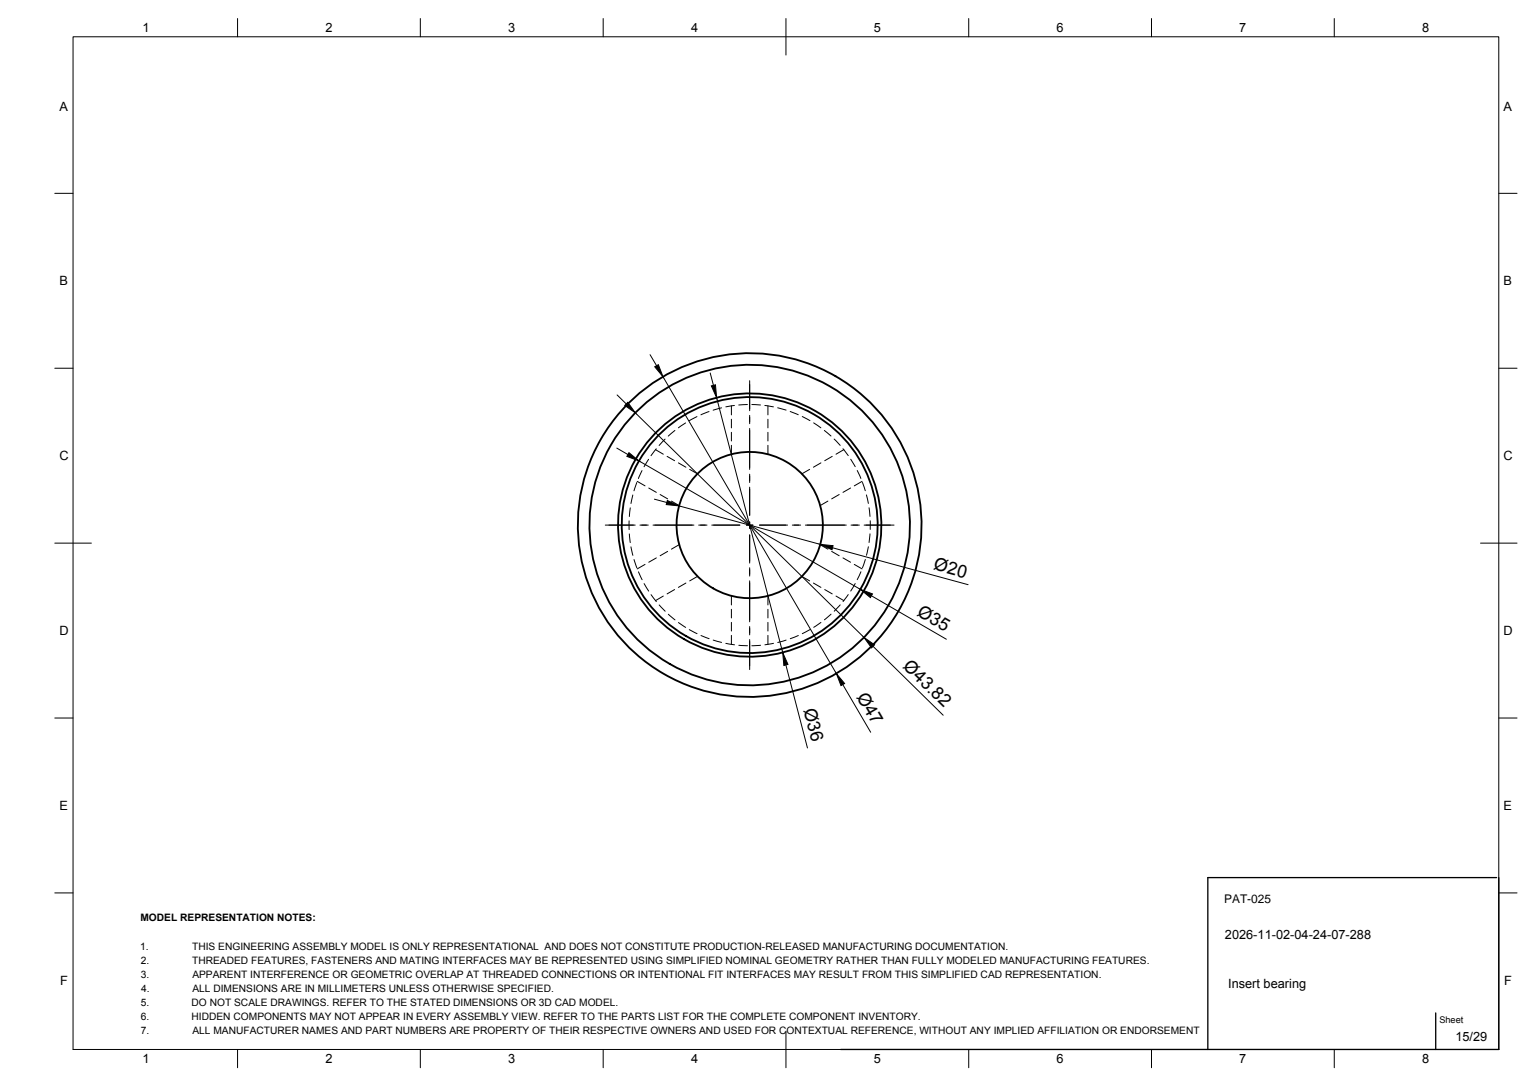
ISO-10303-21;
HEADER;
/* Generated by software containing ST-Developer
 * from STEP Tools, Inc. (www.steptools.com) 
 */

FILE_DESCRIPTION(
/* description */ ('Counter shaft with two pulleys and keyed hub'),
/* implementation_level */ '2;1');

FILE_NAME(
/* name */ 'Insert bearing.step',
/* time_stamp */ '2026-10-27T10:46:10-07:00',
/* author */ (''),
/* organization */ (''),
/* preprocessor_version */ 'ST-DEVELOPER v20.2',
/* originating_system */ 'Autodesk Translation Framework v15.17.0.0',
/* authorisation */ '');

FILE_SCHEMA (('AUTOMOTIVE_DESIGN { 1 0 10303 214 3 1 1 }'));
ENDSEC;

DATA;
#10=MECHANICAL_DESIGN_GEOMETRIC_PRESENTATION_REPRESENTATION('',(#298,#299),#10821);
#184=B_SPLINE_CURVE_WITH_KNOTS('',3,(#8629,#8630,#8631,#8632,#8633,#8634,
#8635,#8636,#8637,#8638),.UNSPECIFIED.,.F.,.F.,(4,2,2,2,4),(1.13193471301885,
1.22626174930539,1.32058878559194,1.41491753480854,1.50924628402513),
 .UNSPECIFIED.);
#185=B_SPLINE_CURVE_WITH_KNOTS('',3,(#8640,#8641,#8642,#8643,#8644,#8645,
#8646,#8647,#8648,#8649,#8650,#8651,#8652,#8653,#8654,#8655,#8656,#8657),
 .UNSPECIFIED.,.F.,.F.,(4,2,2,2,2,2,2,2,4),(0.377311571006283,0.471638607292829,
0.565965643579376,0.66029439279597,0.754623142012565,0.84895189122916,0.943280640445754,
1.0376076767323,1.13193471301885),.UNSPECIFIED.);
#186=B_SPLINE_CURVE_WITH_KNOTS('',3,(#8658,#8659,#8660,#8661,#8662,#8663,
#8664,#8665,#8666,#8667),.UNSPECIFIED.,.F.,.F.,(4,2,2,2,4),(1.50924628402513,
1.60357503324173,1.69790378245832,1.79223081874487,1.88655785503141),
 .UNSPECIFIED.);
#187=B_SPLINE_CURVE_WITH_KNOTS('',3,(#8670,#8671,#8672,#8673,#8674,#8675,
#8676,#8677,#8678,#8679,#8680,#8681,#8682,#8683,#8684,#8685,#8686,#8687,
#8688,#8689,#8690,#8691,#8692,#8693,#8694,#8695,#8696,#8697,#8698,#8699,
#8700,#8701,#8702,#8703),.UNSPECIFIED.,.T.,.F.,(4,2,2,2,2,2,2,2,2,2,2,2,
2,2,2,2,4),(0.,0.0946120580087934,0.189224116017587,0.283822945575014,0.378421775132442,
0.47302060468987,0.567619434247297,0.662231492256091,0.756843550264884,
0.851455608273677,0.94606766628247,1.0406664958399,1.13526532539733,1.22986415495475,
1.32446298451218,1.41907504252097,1.51368710052977),.UNSPECIFIED.);
#188=B_SPLINE_CURVE_WITH_KNOTS('',3,(#8706,#8707,#8708,#8709,#8710,#8711,
#8712,#8713,#8714,#8715,#8716,#8717,#8718,#8719,#8720,#8721,#8722,#8723,
#8724,#8725,#8726,#8727,#8728,#8729,#8730,#8731,#8732,#8733,#8734,#8735,
#8736,#8737,#8738,#8739),.UNSPECIFIED.,.T.,.F.,(4,2,2,2,2,2,2,2,2,2,2,2,
2,2,2,2,4),(0.,0.0946120580087934,0.189224116017587,0.283822945575014,0.378421775132442,
0.47302060468987,0.567619434247297,0.66223149225609,0.756843550264884,0.851455608273677,
0.94606766628247,1.0406664958399,1.13526532539733,1.22986415495475,1.32446298451218,
1.41907504252097,1.51368710052977),.UNSPECIFIED.);
#189=B_SPLINE_CURVE_WITH_KNOTS('',3,(#8743,#8744,#8745,#8746,#8747,#8748,
#8749,#8750,#8751,#8752),.UNSPECIFIED.,.F.,.F.,(4,2,2,2,4),(1.13193471301885,
1.22626174930539,1.32058878559194,1.41491753480854,1.50924628402513),
 .UNSPECIFIED.);
#190=B_SPLINE_CURVE_WITH_KNOTS('',3,(#8754,#8755,#8756,#8757,#8758,#8759,
#8760,#8761,#8762,#8763,#8764,#8765,#8766,#8767,#8768,#8769,#8770,#8771),
 .UNSPECIFIED.,.F.,.F.,(4,2,2,2,2,2,2,2,4),(0.377311571006283,0.47163860729283,
0.565965643579376,0.660294392795971,0.754623142012565,0.84895189122916,
0.943280640445755,1.0376076767323,1.13193471301885),.UNSPECIFIED.);
#191=B_SPLINE_CURVE_WITH_KNOTS('',3,(#8772,#8773,#8774,#8775,#8776,#8777,
#8778,#8779,#8780,#8781),.UNSPECIFIED.,.F.,.F.,(4,2,2,2,4),(1.50924628402513,
1.60357503324173,1.69790378245832,1.79223081874487,1.88655785503141),
 .UNSPECIFIED.);
#192=B_SPLINE_CURVE_WITH_KNOTS('',3,(#8790,#8791,#8792,#8793,#8794,#8795,
#8796,#8797,#8798,#8799,#8800,#8801,#8802,#8803,#8804,#8805,#8806,#8807),
 .UNSPECIFIED.,.F.,.F.,(4,2,2,2,2,2,2,2,4),(0.377311571006282,0.471638607292829,
0.565965643579376,0.660294392795971,0.754623142012565,0.84895189122916,
0.943280640445754,1.0376076767323,1.13193471301885),.UNSPECIFIED.);
#193=B_SPLINE_CURVE_WITH_KNOTS('',3,(#8809,#8810,#8811,#8812,#8813,#8814,
#8815,#8816,#8817,#8818),.UNSPECIFIED.,.F.,.F.,(4,2,2,2,4),(1.13193471301885,
1.22626174930539,1.32058878559194,1.41491753480854,1.50924628402513),
 .UNSPECIFIED.);
#194=B_SPLINE_CURVE_WITH_KNOTS('',3,(#8819,#8820,#8821,#8822,#8823,#8824,
#8825,#8826,#8827,#8828),.UNSPECIFIED.,.F.,.F.,(4,2,2,2,4),(1.50924628402513,
1.60357503324172,1.69790378245832,1.79223081874487,1.88655785503141),
 .UNSPECIFIED.);
#195=B_SPLINE_CURVE_WITH_KNOTS('',3,(#8831,#8832,#8833,#8834,#8835,#8836,
#8837,#8838,#8839,#8840,#8841,#8842,#8843,#8844,#8845,#8846,#8847,#8848),
 .UNSPECIFIED.,.F.,.F.,(4,2,2,2,2,2,2,2,4),(0.377311571006283,0.47163860729283,
0.565965643579376,0.660294392795971,0.754623142012565,0.84895189122916,
0.943280640445754,1.0376076767323,1.13193471301885),.UNSPECIFIED.);
#196=B_SPLINE_CURVE_WITH_KNOTS('',3,(#8850,#8851,#8852,#8853,#8854,#8855,
#8856,#8857,#8858,#8859),.UNSPECIFIED.,.F.,.F.,(4,2,2,2,4),(1.13193471301885,
1.22626174930539,1.32058878559194,1.41491753480854,1.50924628402513),
 .UNSPECIFIED.);
#197=B_SPLINE_CURVE_WITH_KNOTS('',3,(#8860,#8861,#8862,#8863,#8864,#8865,
#8866,#8867,#8868,#8869),.UNSPECIFIED.,.F.,.F.,(4,2,2,2,4),(1.50924628402513,
1.60357503324173,1.69790378245832,1.79223081874487,1.88655785503141),
 .UNSPECIFIED.);
#198=B_SPLINE_CURVE_WITH_KNOTS('',3,(#8872,#8873,#8874,#8875,#8876,#8877,
#8878,#8879,#8880,#8881,#8882,#8883,#8884,#8885,#8886,#8887,#8888,#8889),
 .UNSPECIFIED.,.F.,.F.,(4,2,2,2,2,2,2,2,4),(0.377311571006282,0.471638607292829,
0.565965643579376,0.66029439279597,0.754623142012565,0.84895189122916,0.943280640445754,
1.0376076767323,1.13193471301885),.UNSPECIFIED.);
#199=B_SPLINE_CURVE_WITH_KNOTS('',3,(#8891,#8892,#8893,#8894,#8895,#8896,
#8897,#8898,#8899,#8900),.UNSPECIFIED.,.F.,.F.,(4,2,2,2,4),(1.13193471301885,
1.22626174930539,1.32058878559194,1.41491753480854,1.50924628402513),
 .UNSPECIFIED.);
#200=B_SPLINE_CURVE_WITH_KNOTS('',3,(#8901,#8902,#8903,#8904,#8905,#8906,
#8907,#8908,#8909,#8910),.UNSPECIFIED.,.F.,.F.,(4,2,2,2,4),(1.50924628402513,
1.60357503324172,1.69790378245832,1.79223081874487,1.88655785503141),
 .UNSPECIFIED.);
#201=B_SPLINE_CURVE_WITH_KNOTS('',3,(#8913,#8914,#8915,#8916,#8917,#8918,
#8919,#8920,#8921,#8922,#8923,#8924,#8925,#8926,#8927,#8928,#8929,#8930),
 .UNSPECIFIED.,.F.,.F.,(4,2,2,2,2,2,2,2,4),(0.377311571006283,0.471638607292829,
0.565965643579376,0.660294392795971,0.754623142012565,0.84895189122916,
0.943280640445755,1.0376076767323,1.13193471301885),.UNSPECIFIED.);
#202=B_SPLINE_CURVE_WITH_KNOTS('',3,(#8932,#8933,#8934,#8935,#8936,#8937,
#8938,#8939,#8940,#8941),.UNSPECIFIED.,.F.,.F.,(4,2,2,2,4),(1.13193471301885,
1.22626174930539,1.32058878559194,1.41491753480854,1.50924628402513),
 .UNSPECIFIED.);
#203=B_SPLINE_CURVE_WITH_KNOTS('',3,(#8942,#8943,#8944,#8945,#8946,#8947,
#8948,#8949,#8950,#8951),.UNSPECIFIED.,.F.,.F.,(4,2,2,2,4),(1.50924628402513,
1.60357503324172,1.69790378245832,1.79223081874487,1.88655785503141),
 .UNSPECIFIED.);
#204=B_SPLINE_CURVE_WITH_KNOTS('',3,(#8955,#8956,#8957,#8958,#8959,#8960,
#8961,#8962,#8963,#8964,#8965,#8966,#8967,#8968,#8969,#8970,#8971,#8972,
#8973,#8974,#8975,#8976,#8977,#8978,#8979,#8980,#8981,#8982,#8983,#8984,
#8985,#8986,#8987,#8988),.UNSPECIFIED.,.T.,.F.,(4,2,2,2,2,2,2,2,2,2,2,2,
2,2,2,2,4),(0.,0.0946120580087934,0.189224116017587,0.283822945575014,0.378421775132442,
0.47302060468987,0.567619434247297,0.66223149225609,0.756843550264884,0.851455608273677,
0.94606766628247,1.0406664958399,1.13526532539733,1.22986415495475,1.32446298451218,
1.41907504252097,1.51368710052977),.UNSPECIFIED.);
#205=B_SPLINE_CURVE_WITH_KNOTS('',3,(#8991,#8992,#8993,#8994,#8995,#8996,
#8997,#8998,#8999,#9000,#9001,#9002,#9003,#9004,#9005,#9006,#9007,#9008,
#9009,#9010,#9011,#9012,#9013,#9014,#9015,#9016,#9017,#9018,#9019,#9020,
#9021,#9022,#9023,#9024),.UNSPECIFIED.,.T.,.F.,(4,2,2,2,2,2,2,2,2,2,2,2,
2,2,2,2,4),(0.,0.0946120580087934,0.189224116017587,0.283822945575014,0.378421775132442,
0.47302060468987,0.567619434247297,0.66223149225609,0.756843550264884,0.851455608273677,
0.94606766628247,1.0406664958399,1.13526532539733,1.22986415495475,1.32446298451218,
1.41907504252097,1.51368710052977),.UNSPECIFIED.);
#206=B_SPLINE_CURVE_WITH_KNOTS('',3,(#9029,#9030,#9031,#9032,#9033,#9034,
#9035,#9036,#9037,#9038,#9039,#9040,#9041,#9042,#9043,#9044,#9045,#9046,
#9047,#9048,#9049,#9050,#9051,#9052,#9053,#9054,#9055,#9056,#9057,#9058,
#9059,#9060,#9061,#9062),.UNSPECIFIED.,.T.,.F.,(4,2,2,2,2,2,2,2,2,2,2,2,
2,2,2,2,4),(0.,0.0946120580087934,0.189224116017587,0.283822945575014,0.378421775132442,
0.47302060468987,0.567619434247297,0.66223149225609,0.756843550264884,0.851455608273677,
0.94606766628247,1.0406664958399,1.13526532539733,1.22986415495475,1.32446298451218,
1.41907504252097,1.51368710052977),.UNSPECIFIED.);
#207=B_SPLINE_CURVE_WITH_KNOTS('',3,(#9065,#9066,#9067,#9068,#9069,#9070,
#9071,#9072,#9073,#9074,#9075,#9076,#9077,#9078,#9079,#9080,#9081,#9082,
#9083,#9084,#9085,#9086,#9087,#9088,#9089,#9090,#9091,#9092,#9093,#9094,
#9095,#9096,#9097,#9098),.UNSPECIFIED.,.T.,.F.,(4,2,2,2,2,2,2,2,2,2,2,2,
2,2,2,2,4),(0.,0.0946120580087934,0.189224116017587,0.283822945575014,0.378421775132442,
0.47302060468987,0.567619434247297,0.66223149225609,0.756843550264884,0.851455608273677,
0.94606766628247,1.0406664958399,1.13526532539733,1.22986415495475,1.32446298451218,
1.41907504252097,1.51368710052977),.UNSPECIFIED.);
#239=SPHERICAL_SURFACE('',#5996,2.35);
#248=SHAPE_REPRESENTATION_RELATIONSHIP('SRR','None',#10935,#273);
#273=ADVANCED_BREP_SHAPE_REPRESENTATION('',(#324,#325),#10803);
#298=STYLED_ITEM('',(#11135),#324);
#299=STYLED_ITEM('',(#11135),#325);
#324=MANIFOLD_SOLID_BREP('Body1',#5581);
#325=MANIFOLD_SOLID_BREP('Body2',#5582);
#366=FACE_BOUND('',#993,.T.);
#367=FACE_BOUND('',#995,.T.);
#368=FACE_BOUND('',#996,.T.);
#369=FACE_BOUND('',#998,.T.);
#370=FACE_BOUND('',#1002,.T.);
#371=FACE_BOUND('',#1003,.T.);
#372=FACE_BOUND('',#1004,.T.);
#373=FACE_BOUND('',#1005,.T.);
#374=FACE_BOUND('',#1006,.T.);
#375=FACE_BOUND('',#1007,.T.);
#376=FACE_BOUND('',#1013,.T.);
#377=FACE_BOUND('',#1015,.T.);
#378=FACE_BOUND('',#1018,.T.);
#379=FACE_BOUND('',#1020,.T.);
#380=FACE_BOUND('',#1021,.T.);
#381=FACE_BOUND('',#1022,.T.);
#382=FACE_BOUND('',#1023,.T.);
#383=FACE_BOUND('',#1024,.T.);
#384=FACE_BOUND('',#1025,.T.);
#476=PLANE('',#5994);
#477=PLANE('',#5999);
#478=PLANE('',#6009);
#479=PLANE('',#6011);
#480=PLANE('',#6015);
#651=FACE_OUTER_BOUND('',#991,.T.);
#652=FACE_OUTER_BOUND('',#992,.T.);
#653=FACE_OUTER_BOUND('',#994,.T.);
#654=FACE_OUTER_BOUND('',#997,.T.);
#655=FACE_OUTER_BOUND('',#999,.T.);
#656=FACE_OUTER_BOUND('',#1000,.T.);
#657=FACE_OUTER_BOUND('',#1001,.T.);
#658=FACE_OUTER_BOUND('',#1008,.T.);
#659=FACE_OUTER_BOUND('',#1009,.T.);
#660=FACE_OUTER_BOUND('',#1010,.T.);
#661=FACE_OUTER_BOUND('',#1011,.T.);
#662=FACE_OUTER_BOUND('',#1012,.T.);
#663=FACE_OUTER_BOUND('',#1014,.T.);
#664=FACE_OUTER_BOUND('',#1016,.T.);
#665=FACE_OUTER_BOUND('',#1017,.T.);
#666=FACE_OUTER_BOUND('',#1019,.T.);
#991=EDGE_LOOP('',(#3895,#3896,#3897,#3898));
#992=EDGE_LOOP('',(#3899));
#993=EDGE_LOOP('',(#3900));
#994=EDGE_LOOP('',(#3901,#3902));
#995=EDGE_LOOP('',(#3903));
#996=EDGE_LOOP('',(#3904));
#997=EDGE_LOOP('',(#3905));
#998=EDGE_LOOP('',(#3906));
#999=EDGE_LOOP('',(#3907,#3908,#3909,#3910,#3911,#3912));
#1000=EDGE_LOOP('',(#3913,#3914,#3915,#3916,#3917,#3918));
#1001=EDGE_LOOP('',(#3919,#3920,#3921,#3922));
#1002=EDGE_LOOP('',(#3923,#3924,#3925));
#1003=EDGE_LOOP('',(#3926,#3927,#3928));
#1004=EDGE_LOOP('',(#3929,#3930,#3931));
#1005=EDGE_LOOP('',(#3932,#3933,#3934));
#1006=EDGE_LOOP('',(#3935,#3936,#3937));
#1007=EDGE_LOOP('',(#3938,#3939,#3940));
#1008=EDGE_LOOP('',(#3941,#3942,#3943,#3944,#3945,#3946));
#1009=EDGE_LOOP('',(#3947,#3948,#3949,#3950,#3951,#3952));
#1010=EDGE_LOOP('',(#3953,#3954,#3955,#3956,#3957,#3958));
#1011=EDGE_LOOP('',(#3959,#3960,#3961,#3962,#3963,#3964));
#1012=EDGE_LOOP('',(#3965));
#1013=EDGE_LOOP('',(#3966));
#1014=EDGE_LOOP('',(#3967));
#1015=EDGE_LOOP('',(#3968));
#1016=EDGE_LOOP('',(#3969,#3970,#3971,#3972));
#1017=EDGE_LOOP('',(#3973));
#1018=EDGE_LOOP('',(#3974));
#1019=EDGE_LOOP('',(#3975,#3976,#3977,#3978));
#1020=EDGE_LOOP('',(#3979));
#1021=EDGE_LOOP('',(#3980));
#1022=EDGE_LOOP('',(#3981));
#1023=EDGE_LOOP('',(#3982));
#1024=EDGE_LOOP('',(#3983));
#1025=EDGE_LOOP('',(#3984));
#1401=LINE('',#8614,#1790);
#1402=LINE('',#8669,#1791);
#1403=LINE('',#8741,#1792);
#1404=LINE('',#8786,#1793);
#1405=LINE('',#8954,#1794);
#1406=LINE('',#9025,#1795);
#1407=LINE('',#9028,#1796);
#1408=LINE('',#9099,#1797);
#1409=LINE('',#9109,#1798);
#1410=LINE('',#9114,#1799);
#1790=VECTOR('',#6885,1.8);
#1791=VECTOR('',#6902,0.25);
#1792=VECTOR('',#6905,0.25);
#1793=VECTOR('',#6910,1.65);
#1794=VECTOR('',#6915,0.25);
#1795=VECTOR('',#6918,0.25);
#1796=VECTOR('',#6921,0.25);
#1797=VECTOR('',#6924,0.25);
#1798=VECTOR('',#6937,1.75);
#1799=VECTOR('',#6944,1.);
#2124=CIRCLE('',#5992,1.8);
#2125=CIRCLE('',#5993,1.8);
#2126=CIRCLE('',#5995,2.19089023002066);
#2127=CIRCLE('',#5997,2.35);
#2128=CIRCLE('',#5998,2.19089023002066);
#2129=CIRCLE('',#6003,1.65);
#2130=CIRCLE('',#6004,1.65);
#2131=CIRCLE('',#6010,1.);
#2132=CIRCLE('',#6012,1.75);
#2133=CIRCLE('',#6014,1.75);
#2134=CIRCLE('',#6016,1.);
#2474=VERTEX_POINT('',#8611);
#2475=VERTEX_POINT('',#8613);
#2476=VERTEX_POINT('',#8617);
#2477=VERTEX_POINT('',#8620);
#2478=VERTEX_POINT('',#8621);
#2479=VERTEX_POINT('',#8623);
#2480=VERTEX_POINT('',#8627);
#2481=VERTEX_POINT('',#8628);
#2482=VERTEX_POINT('',#8639);
#2483=VERTEX_POINT('',#8668);
#2484=VERTEX_POINT('',#8705);
#2485=VERTEX_POINT('',#8740);
#2486=VERTEX_POINT('',#8742);
#2487=VERTEX_POINT('',#8753);
#2488=VERTEX_POINT('',#8783);
#2489=VERTEX_POINT('',#8785);
#2490=VERTEX_POINT('',#8788);
#2491=VERTEX_POINT('',#8789);
#2492=VERTEX_POINT('',#8808);
#2493=VERTEX_POINT('',#8829);
#2494=VERTEX_POINT('',#8830);
#2495=VERTEX_POINT('',#8849);
#2496=VERTEX_POINT('',#8870);
#2497=VERTEX_POINT('',#8871);
#2498=VERTEX_POINT('',#8890);
#2499=VERTEX_POINT('',#8911);
#2500=VERTEX_POINT('',#8912);
#2501=VERTEX_POINT('',#8931);
#2502=VERTEX_POINT('',#8953);
#2503=VERTEX_POINT('',#8990);
#2504=VERTEX_POINT('',#9027);
#2505=VERTEX_POINT('',#9064);
#2506=VERTEX_POINT('',#9101);
#2507=VERTEX_POINT('',#9104);
#2508=VERTEX_POINT('',#9107);
#2509=VERTEX_POINT('',#9111);
#3020=EDGE_CURVE('',#2474,#2474,#2124,.T.);
#3021=EDGE_CURVE('',#2474,#2475,#1401,.T.);
#3022=EDGE_CURVE('',#2475,#2475,#2125,.T.);
#3023=EDGE_CURVE('',#2476,#2476,#2126,.T.);
#3024=EDGE_CURVE('',#2477,#2478,#2127,.T.);
#3025=EDGE_CURVE('',#2479,#2479,#2128,.T.);
#3026=EDGE_CURVE('',#2480,#2481,#184,.T.);
#3027=EDGE_CURVE('',#2482,#2480,#185,.T.);
#3028=EDGE_CURVE('',#2481,#2482,#186,.T.);
#3029=EDGE_CURVE('',#2481,#2483,#1402,.T.);
#3030=EDGE_CURVE('',#2483,#2483,#187,.T.);
#3031=EDGE_CURVE('',#2484,#2484,#188,.T.);
#3032=EDGE_CURVE('',#2484,#2485,#1403,.T.);
#3033=EDGE_CURVE('',#2486,#2485,#189,.T.);
#3034=EDGE_CURVE('',#2487,#2486,#190,.T.);
#3035=EDGE_CURVE('',#2485,#2487,#191,.T.);
#3036=EDGE_CURVE('',#2488,#2488,#2129,.T.);
#3037=EDGE_CURVE('',#2488,#2489,#1404,.T.);
#3038=EDGE_CURVE('',#2489,#2489,#2130,.T.);
#3039=EDGE_CURVE('',#2490,#2491,#192,.T.);
#3040=EDGE_CURVE('',#2491,#2492,#193,.T.);
#3041=EDGE_CURVE('',#2492,#2490,#194,.T.);
#3042=EDGE_CURVE('',#2493,#2494,#195,.T.);
#3043=EDGE_CURVE('',#2494,#2495,#196,.T.);
#3044=EDGE_CURVE('',#2495,#2493,#197,.T.);
#3045=EDGE_CURVE('',#2496,#2497,#198,.T.);
#3046=EDGE_CURVE('',#2497,#2498,#199,.T.);
#3047=EDGE_CURVE('',#2498,#2496,#200,.T.);
#3048=EDGE_CURVE('',#2499,#2500,#201,.T.);
#3049=EDGE_CURVE('',#2500,#2501,#202,.T.);
#3050=EDGE_CURVE('',#2501,#2499,#203,.T.);
#3051=EDGE_CURVE('',#2492,#2502,#1405,.T.);
#3052=EDGE_CURVE('',#2502,#2502,#204,.T.);
#3053=EDGE_CURVE('',#2503,#2503,#205,.T.);
#3054=EDGE_CURVE('',#2503,#2495,#1406,.T.);
#3055=EDGE_CURVE('',#2498,#2504,#1407,.T.);
#3056=EDGE_CURVE('',#2504,#2504,#206,.T.);
#3057=EDGE_CURVE('',#2505,#2505,#207,.T.);
#3058=EDGE_CURVE('',#2505,#2501,#1408,.T.);
#3059=EDGE_CURVE('',#2506,#2506,#2131,.T.);
#3060=EDGE_CURVE('',#2507,#2507,#2132,.T.);
#3061=EDGE_CURVE('',#2508,#2508,#2133,.T.);
#3062=EDGE_CURVE('',#2508,#2507,#1409,.T.);
#3063=EDGE_CURVE('',#2509,#2509,#2134,.T.);
#3064=EDGE_CURVE('',#2509,#2506,#1410,.T.);
#3895=ORIENTED_EDGE('',*,*,#3020,.T.);
#3896=ORIENTED_EDGE('',*,*,#3021,.T.);
#3897=ORIENTED_EDGE('',*,*,#3022,.F.);
#3898=ORIENTED_EDGE('',*,*,#3021,.F.);
#3899=ORIENTED_EDGE('',*,*,#3023,.F.);
#3900=ORIENTED_EDGE('',*,*,#3022,.T.);
#3901=ORIENTED_EDGE('',*,*,#3024,.T.);
#3902=ORIENTED_EDGE('',*,*,#3024,.F.);
#3903=ORIENTED_EDGE('',*,*,#3023,.T.);
#3904=ORIENTED_EDGE('',*,*,#3025,.F.);
#3905=ORIENTED_EDGE('',*,*,#3025,.T.);
#3906=ORIENTED_EDGE('',*,*,#3020,.F.);
#3907=ORIENTED_EDGE('',*,*,#3026,.F.);
#3908=ORIENTED_EDGE('',*,*,#3027,.F.);
#3909=ORIENTED_EDGE('',*,*,#3028,.F.);
#3910=ORIENTED_EDGE('',*,*,#3029,.T.);
#3911=ORIENTED_EDGE('',*,*,#3030,.F.);
#3912=ORIENTED_EDGE('',*,*,#3029,.F.);
#3913=ORIENTED_EDGE('',*,*,#3031,.F.);
#3914=ORIENTED_EDGE('',*,*,#3032,.T.);
#3915=ORIENTED_EDGE('',*,*,#3033,.F.);
#3916=ORIENTED_EDGE('',*,*,#3034,.F.);
#3917=ORIENTED_EDGE('',*,*,#3035,.F.);
#3918=ORIENTED_EDGE('',*,*,#3032,.F.);
#3919=ORIENTED_EDGE('',*,*,#3036,.F.);
#3920=ORIENTED_EDGE('',*,*,#3037,.T.);
#3921=ORIENTED_EDGE('',*,*,#3038,.T.);
#3922=ORIENTED_EDGE('',*,*,#3037,.F.);
#3923=ORIENTED_EDGE('',*,*,#3027,.T.);
#3924=ORIENTED_EDGE('',*,*,#3026,.T.);
#3925=ORIENTED_EDGE('',*,*,#3028,.T.);
#3926=ORIENTED_EDGE('',*,*,#3034,.T.);
#3927=ORIENTED_EDGE('',*,*,#3033,.T.);
#3928=ORIENTED_EDGE('',*,*,#3035,.T.);
#3929=ORIENTED_EDGE('',*,*,#3039,.T.);
#3930=ORIENTED_EDGE('',*,*,#3040,.T.);
#3931=ORIENTED_EDGE('',*,*,#3041,.T.);
#3932=ORIENTED_EDGE('',*,*,#3042,.T.);
#3933=ORIENTED_EDGE('',*,*,#3043,.T.);
#3934=ORIENTED_EDGE('',*,*,#3044,.T.);
#3935=ORIENTED_EDGE('',*,*,#3045,.T.);
#3936=ORIENTED_EDGE('',*,*,#3046,.T.);
#3937=ORIENTED_EDGE('',*,*,#3047,.T.);
#3938=ORIENTED_EDGE('',*,*,#3048,.T.);
#3939=ORIENTED_EDGE('',*,*,#3049,.T.);
#3940=ORIENTED_EDGE('',*,*,#3050,.T.);
#3941=ORIENTED_EDGE('',*,*,#3040,.F.);
#3942=ORIENTED_EDGE('',*,*,#3039,.F.);
#3943=ORIENTED_EDGE('',*,*,#3041,.F.);
#3944=ORIENTED_EDGE('',*,*,#3051,.T.);
#3945=ORIENTED_EDGE('',*,*,#3052,.F.);
#3946=ORIENTED_EDGE('',*,*,#3051,.F.);
#3947=ORIENTED_EDGE('',*,*,#3053,.F.);
#3948=ORIENTED_EDGE('',*,*,#3054,.T.);
#3949=ORIENTED_EDGE('',*,*,#3043,.F.);
#3950=ORIENTED_EDGE('',*,*,#3042,.F.);
#3951=ORIENTED_EDGE('',*,*,#3044,.F.);
#3952=ORIENTED_EDGE('',*,*,#3054,.F.);
#3953=ORIENTED_EDGE('',*,*,#3046,.F.);
#3954=ORIENTED_EDGE('',*,*,#3045,.F.);
#3955=ORIENTED_EDGE('',*,*,#3047,.F.);
#3956=ORIENTED_EDGE('',*,*,#3055,.T.);
#3957=ORIENTED_EDGE('',*,*,#3056,.F.);
#3958=ORIENTED_EDGE('',*,*,#3055,.F.);
#3959=ORIENTED_EDGE('',*,*,#3057,.F.);
#3960=ORIENTED_EDGE('',*,*,#3058,.T.);
#3961=ORIENTED_EDGE('',*,*,#3049,.F.);
#3962=ORIENTED_EDGE('',*,*,#3048,.F.);
#3963=ORIENTED_EDGE('',*,*,#3050,.F.);
#3964=ORIENTED_EDGE('',*,*,#3058,.F.);
#3965=ORIENTED_EDGE('',*,*,#3038,.F.);
#3966=ORIENTED_EDGE('',*,*,#3059,.T.);
#3967=ORIENTED_EDGE('',*,*,#3060,.F.);
#3968=ORIENTED_EDGE('',*,*,#3036,.T.);
#3969=ORIENTED_EDGE('',*,*,#3061,.F.);
#3970=ORIENTED_EDGE('',*,*,#3062,.T.);
#3971=ORIENTED_EDGE('',*,*,#3060,.T.);
#3972=ORIENTED_EDGE('',*,*,#3062,.F.);
#3973=ORIENTED_EDGE('',*,*,#3061,.T.);
#3974=ORIENTED_EDGE('',*,*,#3063,.F.);
#3975=ORIENTED_EDGE('',*,*,#3063,.T.);
#3976=ORIENTED_EDGE('',*,*,#3064,.T.);
#3977=ORIENTED_EDGE('',*,*,#3059,.F.);
#3978=ORIENTED_EDGE('',*,*,#3064,.F.);
#3979=ORIENTED_EDGE('',*,*,#3031,.T.);
#3980=ORIENTED_EDGE('',*,*,#3030,.T.);
#3981=ORIENTED_EDGE('',*,*,#3053,.T.);
#3982=ORIENTED_EDGE('',*,*,#3052,.T.);
#3983=ORIENTED_EDGE('',*,*,#3057,.T.);
#3984=ORIENTED_EDGE('',*,*,#3056,.T.);
#5130=CYLINDRICAL_SURFACE('',#5991,1.8);
#5131=CYLINDRICAL_SURFACE('',#6000,0.25);
#5132=CYLINDRICAL_SURFACE('',#6001,0.25);
#5133=CYLINDRICAL_SURFACE('',#6002,1.65);
#5134=CYLINDRICAL_SURFACE('',#6005,0.25);
#5135=CYLINDRICAL_SURFACE('',#6006,0.25);
#5136=CYLINDRICAL_SURFACE('',#6007,0.25);
#5137=CYLINDRICAL_SURFACE('',#6008,0.25);
#5138=CYLINDRICAL_SURFACE('',#6013,1.75);
#5139=CYLINDRICAL_SURFACE('',#6017,1.);
#5322=ADVANCED_FACE('',(#651),#5130,.F.);
#5323=ADVANCED_FACE('',(#652,#366),#476,.T.);
#5324=ADVANCED_FACE('',(#653,#367,#368),#239,.T.);
#5325=ADVANCED_FACE('',(#654,#369),#477,.T.);
#5326=ADVANCED_FACE('',(#655),#5131,.F.);
#5327=ADVANCED_FACE('',(#656),#5132,.F.);
#5328=ADVANCED_FACE('',(#657,#370,#371,#372,#373,#374,#375),#5133,.T.);
#5329=ADVANCED_FACE('',(#658),#5134,.F.);
#5330=ADVANCED_FACE('',(#659),#5135,.F.);
#5331=ADVANCED_FACE('',(#660),#5136,.F.);
#5332=ADVANCED_FACE('',(#661),#5137,.F.);
#5333=ADVANCED_FACE('',(#662,#376),#478,.T.);
#5334=ADVANCED_FACE('',(#663,#377),#479,.T.);
#5335=ADVANCED_FACE('',(#664),#5138,.T.);
#5336=ADVANCED_FACE('',(#665,#378),#480,.T.);
#5337=ADVANCED_FACE('',(#666,#379,#380,#381,#382,#383,#384),#5139,.F.);
#5581=CLOSED_SHELL('',(#5322,#5323,#5324,#5325));
#5582=CLOSED_SHELL('',(#5326,#5327,#5328,#5329,#5330,#5331,#5332,#5333,
#5334,#5335,#5336,#5337));
#5990=AXIS2_PLACEMENT_3D('',#8609,#6879,#6880);
#5991=AXIS2_PLACEMENT_3D('',#8610,#6881,#6882);
#5992=AXIS2_PLACEMENT_3D('',#8612,#6883,#6884);
#5993=AXIS2_PLACEMENT_3D('',#8615,#6886,#6887);
#5994=AXIS2_PLACEMENT_3D('',#8616,#6888,#6889);
#5995=AXIS2_PLACEMENT_3D('',#8618,#6890,#6891);
#5996=AXIS2_PLACEMENT_3D('',#8619,#6892,#6893);
#5997=AXIS2_PLACEMENT_3D('',#8622,#6894,#6895);
#5998=AXIS2_PLACEMENT_3D('',#8624,#6896,#6897);
#5999=AXIS2_PLACEMENT_3D('',#8625,#6898,#6899);
#6000=AXIS2_PLACEMENT_3D('',#8626,#6900,#6901);
#6001=AXIS2_PLACEMENT_3D('',#8704,#6903,#6904);
#6002=AXIS2_PLACEMENT_3D('',#8782,#6906,#6907);
#6003=AXIS2_PLACEMENT_3D('',#8784,#6908,#6909);
#6004=AXIS2_PLACEMENT_3D('',#8787,#6911,#6912);
#6005=AXIS2_PLACEMENT_3D('',#8952,#6913,#6914);
#6006=AXIS2_PLACEMENT_3D('',#8989,#6916,#6917);
#6007=AXIS2_PLACEMENT_3D('',#9026,#6919,#6920);
#6008=AXIS2_PLACEMENT_3D('',#9063,#6922,#6923);
#6009=AXIS2_PLACEMENT_3D('',#9100,#6925,#6926);
#6010=AXIS2_PLACEMENT_3D('',#9102,#6927,#6928);
#6011=AXIS2_PLACEMENT_3D('',#9103,#6929,#6930);
#6012=AXIS2_PLACEMENT_3D('',#9105,#6931,#6932);
#6013=AXIS2_PLACEMENT_3D('',#9106,#6933,#6934);
#6014=AXIS2_PLACEMENT_3D('',#9108,#6935,#6936);
#6015=AXIS2_PLACEMENT_3D('',#9110,#6938,#6939);
#6016=AXIS2_PLACEMENT_3D('',#9112,#6940,#6941);
#6017=AXIS2_PLACEMENT_3D('',#9113,#6942,#6943);
#6879=DIRECTION('axis',(0.,0.,1.));
#6880=DIRECTION('refdir',(1.,0.,0.));
#6881=DIRECTION('center_axis',(0.,-1.,0.));
#6882=DIRECTION('ref_axis',(1.,0.,0.));
#6883=DIRECTION('center_axis',(0.,-1.,0.));
#6884=DIRECTION('ref_axis',(1.,0.,0.));
#6885=DIRECTION('',(0.,1.,0.));
#6886=DIRECTION('center_axis',(0.,-1.,0.));
#6887=DIRECTION('ref_axis',(1.,0.,0.));
#6888=DIRECTION('center_axis',(0.,1.,0.));
#6889=DIRECTION('ref_axis',(0.,0.,1.));
#6890=DIRECTION('center_axis',(0.,-1.,0.));
#6891=DIRECTION('ref_axis',(1.,0.,0.));
#6892=DIRECTION('center_axis',(6.12323399573677E-17,0.,1.));
#6893=DIRECTION('ref_axis',(1.,0.,0.));
#6894=DIRECTION('center_axis',(1.22464679914735E-16,-1.,0.));
#6895=DIRECTION('ref_axis',(-1.,-1.22464679914735E-16,0.));
#6896=DIRECTION('center_axis',(0.,-1.,0.));
#6897=DIRECTION('ref_axis',(1.,0.,0.));
#6898=DIRECTION('center_axis',(0.,-1.,0.));
#6899=DIRECTION('ref_axis',(0.,0.,-1.));
#6900=DIRECTION('center_axis',(-0.866025403784438,0.,-0.5));
#6901=DIRECTION('ref_axis',(-0.5,0.,0.866025403784438));
#6902=DIRECTION('',(-0.866025403784438,0.,-0.5));
#6903=DIRECTION('center_axis',(-0.866025403784438,0.,-0.5));
#6904=DIRECTION('ref_axis',(-0.5,0.,0.866025403784438));
#6905=DIRECTION('',(-0.866025403784438,0.,-0.5));
#6906=DIRECTION('center_axis',(0.,-1.,0.));
#6907=DIRECTION('ref_axis',(1.,0.,0.));
#6908=DIRECTION('center_axis',(0.,-1.,0.));
#6909=DIRECTION('ref_axis',(1.,0.,0.));
#6910=DIRECTION('',(0.,1.,0.));
#6911=DIRECTION('center_axis',(0.,-1.,0.));
#6912=DIRECTION('ref_axis',(1.,0.,0.));
#6913=DIRECTION('center_axis',(0.866025403784439,0.,-0.5));
#6914=DIRECTION('ref_axis',(-0.5,0.,-0.866025403784439));
#6915=DIRECTION('',(0.866025403784439,0.,-0.5));
#6916=DIRECTION('center_axis',(0.866025403784439,0.,-0.5));
#6917=DIRECTION('ref_axis',(-0.5,0.,-0.866025403784439));
#6918=DIRECTION('',(0.866025403784439,0.,-0.5));
#6919=DIRECTION('center_axis',(0.,0.,1.));
#6920=DIRECTION('ref_axis',(1.,0.,0.));
#6921=DIRECTION('',(0.,0.,1.));
#6922=DIRECTION('center_axis',(0.,0.,1.));
#6923=DIRECTION('ref_axis',(1.,0.,0.));
#6924=DIRECTION('',(0.,0.,1.));
#6925=DIRECTION('center_axis',(0.,1.,0.));
#6926=DIRECTION('ref_axis',(0.,0.,1.));
#6927=DIRECTION('center_axis',(0.,-1.,0.));
#6928=DIRECTION('ref_axis',(1.,0.,0.));
#6929=DIRECTION('center_axis',(0.,1.,0.));
#6930=DIRECTION('ref_axis',(0.,0.,1.));
#6931=DIRECTION('center_axis',(0.,-1.,0.));
#6932=DIRECTION('ref_axis',(1.,0.,0.));
#6933=DIRECTION('center_axis',(0.,-1.,0.));
#6934=DIRECTION('ref_axis',(1.,0.,0.));
#6935=DIRECTION('center_axis',(0.,-1.,0.));
#6936=DIRECTION('ref_axis',(1.,0.,0.));
#6937=DIRECTION('',(0.,1.,0.));
#6938=DIRECTION('center_axis',(0.,-1.,0.));
#6939=DIRECTION('ref_axis',(0.,0.,-1.));
#6940=DIRECTION('center_axis',(0.,-1.,0.));
#6941=DIRECTION('ref_axis',(1.,0.,0.));
#6942=DIRECTION('center_axis',(0.,-1.,0.));
#6943=DIRECTION('ref_axis',(1.,0.,0.));
#6944=DIRECTION('',(0.,1.,0.));
#8609=CARTESIAN_POINT('',(0.,0.,0.));
#8610=CARTESIAN_POINT('Origin',(0.,0.,0.));
#8611=CARTESIAN_POINT('',(-1.8,-0.85,-2.20436423846524E-16));
#8612=CARTESIAN_POINT('Origin',(0.,-0.85,0.));
#8613=CARTESIAN_POINT('',(-1.8,0.85,-2.20436423846524E-16));
#8614=CARTESIAN_POINT('',(-1.8,0.,-2.20436423846524E-16));
#8615=CARTESIAN_POINT('Origin',(0.,0.85,0.));
#8616=CARTESIAN_POINT('Origin',(2.19089023002066,0.85,0.));
#8617=CARTESIAN_POINT('',(2.19089023002066,0.85,0.));
#8618=CARTESIAN_POINT('Origin',(0.,0.85,0.));
#8619=CARTESIAN_POINT('Origin',(3.99680288865056E-15,0.,0.));
#8620=CARTESIAN_POINT('',(3.85290688975075E-15,-1.76221774462768E-32,2.35));
#8621=CARTESIAN_POINT('',(3.85290688975075E-15,-1.76221774462768E-32,-2.35));
#8622=CARTESIAN_POINT('Origin',(3.99680288865056E-15,0.,0.));
#8623=CARTESIAN_POINT('',(2.19089023002066,-0.85,0.));
#8624=CARTESIAN_POINT('Origin',(0.,-0.85,0.));
#8625=CARTESIAN_POINT('Origin',(1.8,-0.85,0.));
#8626=CARTESIAN_POINT('Origin',(0.,1.55,0.));
#8627=CARTESIAN_POINT('',(1.42894191624432,1.8,0.825000000000001));
#8628=CARTESIAN_POINT('',(1.53744468918255,1.55,0.598968970568896));
#8629=CARTESIAN_POINT('Ctrl Pts',(1.42894191624432,1.8,0.825000000000001));
#8630=CARTESIAN_POINT('Ctrl Pts',(1.44466308895875,1.8,0.797770130104052));
#8631=CARTESIAN_POINT('Ctrl Pts',(1.46055812562105,1.79370633789704,0.768258557763732));
#8632=CARTESIAN_POINT('Ctrl Pts',(1.48824888379079,1.76817777258318,0.713138492740816));
#8633=CARTESIAN_POINT('Ctrl Pts',(1.50008999307766,1.74894552961493,0.687551581002689));
#8634=CARTESIAN_POINT('Ctrl Pts',(1.51812136280714,1.70460745840382,0.646764802471699));
#8635=CARTESIAN_POINT('Ctrl Pts',(1.52552758004446,1.67652816181843,0.628833667319578));
#8636=CARTESIAN_POINT('Ctrl Pts',(1.53516661651472,1.61494799959182,0.604921184808251));
#8637=CARTESIAN_POINT('Ctrl Pts',(1.53744468918255,1.58144291640553,0.598968970568896));
#8638=CARTESIAN_POINT('Ctrl Pts',(1.53744468918255,1.55,0.598968970568896));
#8639=CARTESIAN_POINT('',(1.42894191624432,1.3,0.825000000000001));
#8640=CARTESIAN_POINT('Ctrl Pts',(1.42894191624432,1.3,0.825000000000001));
#8641=CARTESIAN_POINT('Ctrl Pts',(1.4132207435299,1.3,0.852229869895949));
#8642=CARTESIAN_POINT('Ctrl Pts',(1.39561049050871,1.30629366210296,0.880751161609749));
#8643=CARTESIAN_POINT('Ctrl Pts',(1.36172049302549,1.33182222741682,0.932292094146256));
#8644=CARTESIAN_POINT('Ctrl Pts',(1.34548213209931,1.35105447038507,0.955340251466734));
#8645=CARTESIAN_POINT('Ctrl Pts',(1.31917543061769,1.39539254159618,0.99134926498299));
#8646=CARTESIAN_POINT('Ctrl Pts',(1.30734972067592,1.42347183818157,1.00672880483252));
#8647=CARTESIAN_POINT('Ctrl Pts',(1.29146042158868,1.48505200040818,1.02703269653942));
#8648=CARTESIAN_POINT('Ctrl Pts',(1.28744468918255,1.51855708359447,1.03198167246111));
#8649=CARTESIAN_POINT('Ctrl Pts',(1.28744468918255,1.58144291640553,1.03198167246111));
#8650=CARTESIAN_POINT('Ctrl Pts',(1.29146042158868,1.61494799959182,1.02703269653942));
#8651=CARTESIAN_POINT('Ctrl Pts',(1.30734972067592,1.67652816181843,1.00672880483252));
#8652=CARTESIAN_POINT('Ctrl Pts',(1.31917543061769,1.70460745840382,0.991349264982991));
#8653=CARTESIAN_POINT('Ctrl Pts',(1.34548213209931,1.74894552961493,0.955340251466735));
#8654=CARTESIAN_POINT('Ctrl Pts',(1.36172049302549,1.76817777258318,0.932292094146256));
#8655=CARTESIAN_POINT('Ctrl Pts',(1.39561049050871,1.79370633789704,0.880751161609749));
#8656=CARTESIAN_POINT('Ctrl Pts',(1.4132207435299,1.8,0.85222986989595));
#8657=CARTESIAN_POINT('Ctrl Pts',(1.42894191624432,1.8,0.825000000000001));
#8658=CARTESIAN_POINT('Ctrl Pts',(1.53744468918255,1.55,0.598968970568896));
#8659=CARTESIAN_POINT('Ctrl Pts',(1.53744468918255,1.51855708359447,0.598968970568896));
#8660=CARTESIAN_POINT('Ctrl Pts',(1.53516661651472,1.48505200040818,0.60492118480825));
#8661=CARTESIAN_POINT('Ctrl Pts',(1.52552758004446,1.42347183818157,0.628833667319578));
#8662=CARTESIAN_POINT('Ctrl Pts',(1.51812136280714,1.39539254159618,0.646764802471699));
#8663=CARTESIAN_POINT('Ctrl Pts',(1.50008999307766,1.35105447038507,0.687551581002689));
#8664=CARTESIAN_POINT('Ctrl Pts',(1.48824888379079,1.33182222741682,0.713138492740816));
#8665=CARTESIAN_POINT('Ctrl Pts',(1.46055812562105,1.30629366210296,0.768258557763732));
#8666=CARTESIAN_POINT('Ctrl Pts',(1.44466308895875,1.3,0.797770130104052));
#8667=CARTESIAN_POINT('Ctrl Pts',(1.42894191624432,1.3,0.825000000000001));
#8668=CARTESIAN_POINT('',(0.963525491562421,1.55,0.267616567329818));
#8669=CARTESIAN_POINT('',(0.125,1.55,-0.21650635094611));
#8670=CARTESIAN_POINT('Ctrl Pts',(0.963525491562421,1.55,0.267616567329818));
#8671=CARTESIAN_POINT('Ctrl Pts',(0.963525491562421,1.5815373526696,0.267616567329818));
#8672=CARTESIAN_POINT('Ctrl Pts',(0.961833761492987,1.61508042700263,0.273949373987484));
#8673=CARTESIAN_POINT('Ctrl Pts',(0.954308486908894,1.67663267125761,0.299111603474268));
#8674=CARTESIAN_POINT('Ctrl Pts',(0.948394987258249,1.70465411363682,0.31788699900678));
#8675=CARTESIAN_POINT('Ctrl Pts',(0.933155485613026,1.74889618382539,0.360174810895352));
#8676=CARTESIAN_POINT('Ctrl Pts',(0.92278792026947,1.76811531482682,0.386546956384144));
#8677=CARTESIAN_POINT('Ctrl Pts',(0.897143218189782,1.79367084275751,0.442820664919227));
#8678=CARTESIAN_POINT('Ctrl Pts',(0.881791875377343,1.8,0.472691670144998));
#8679=CARTESIAN_POINT('Ctrl Pts',(0.850258932191534,1.8,0.527308329855003));
#8680=CARTESIAN_POINT('Ctrl Pts',(0.832065554235658,1.79367084275751,0.555538485325664));
#8681=CARTESIAN_POINT('Ctrl Pts',(0.796153444118959,1.76811531482682,0.605884303066698));
#8682=CARTESIAN_POINT('Ctrl Pts',(0.778498278845144,1.74889618382539,0.62804895077401));
#8683=CARTESIAN_POINT('Ctrl Pts',(0.749495710301794,1.70465411363682,0.662390652284073));
#8684=CARTESIAN_POINT('Ctrl Pts',(0.73619249062986,1.67663267125761,0.676899590973058));
#8685=CARTESIAN_POINT('Ctrl Pts',(0.718163997970498,1.61508042700263,0.695997784676728));
#8686=CARTESIAN_POINT('Ctrl Pts',(0.713525491562421,1.5815373526696,0.700629269222037));
#8687=CARTESIAN_POINT('Ctrl Pts',(0.713525491562421,1.5184626473304,0.700629269222037));
#8688=CARTESIAN_POINT('Ctrl Pts',(0.718163997970498,1.48491957299737,0.695997784676728));
#8689=CARTESIAN_POINT('Ctrl Pts',(0.73619249062986,1.42336732874239,0.676899590973058));
#8690=CARTESIAN_POINT('Ctrl Pts',(0.749495710301794,1.39534588636318,0.662390652284073));
#8691=CARTESIAN_POINT('Ctrl Pts',(0.778498278845144,1.35110381617461,0.62804895077401));
#8692=CARTESIAN_POINT('Ctrl Pts',(0.796153444118959,1.33188468517318,0.605884303066698));
#8693=CARTESIAN_POINT('Ctrl Pts',(0.832065554235658,1.30632915724249,0.555538485325664));
#8694=CARTESIAN_POINT('Ctrl Pts',(0.850258932191534,1.3,0.527308329855003));
#8695=CARTESIAN_POINT('Ctrl Pts',(0.881791875377343,1.3,0.472691670144998));
#8696=CARTESIAN_POINT('Ctrl Pts',(0.897143218189782,1.30632915724249,0.442820664919227));
#8697=CARTESIAN_POINT('Ctrl Pts',(0.92278792026947,1.33188468517318,0.386546956384144));
#8698=CARTESIAN_POINT('Ctrl Pts',(0.933155485613026,1.35110381617461,0.360174810895352));
#8699=CARTESIAN_POINT('Ctrl Pts',(0.948394987258249,1.39534588636318,0.31788699900678));
#8700=CARTESIAN_POINT('Ctrl Pts',(0.954308486908894,1.42336732874239,0.299111603474268));
#8701=CARTESIAN_POINT('Ctrl Pts',(0.961833761492987,1.48491957299738,0.273949373987484));
#8702=CARTESIAN_POINT('Ctrl Pts',(0.963525491562421,1.5184626473304,0.267616567329818));
#8703=CARTESIAN_POINT('Ctrl Pts',(0.963525491562421,1.55,0.267616567329818));
#8704=CARTESIAN_POINT('Origin',(0.,1.55,0.));
#8705=CARTESIAN_POINT('',(-0.713525491562421,1.55,-0.700629269222037));
#8706=CARTESIAN_POINT('Ctrl Pts',(-0.713525491562421,1.55,-0.700629269222037));
#8707=CARTESIAN_POINT('Ctrl Pts',(-0.713525491562421,1.5184626473304,-0.700629269222037));
#8708=CARTESIAN_POINT('Ctrl Pts',(-0.718163997970498,1.48491957299737,-0.695997784676728));
#8709=CARTESIAN_POINT('Ctrl Pts',(-0.73619249062986,1.42336732874239,-0.676899590973058));
#8710=CARTESIAN_POINT('Ctrl Pts',(-0.749495710301794,1.39534588636318,-0.662390652284073));
#8711=CARTESIAN_POINT('Ctrl Pts',(-0.778498278845144,1.35110381617461,-0.62804895077401));
#8712=CARTESIAN_POINT('Ctrl Pts',(-0.796153444118959,1.33188468517318,-0.605884303066698));
#8713=CARTESIAN_POINT('Ctrl Pts',(-0.832065554235658,1.30632915724249,-0.555538485325664));
#8714=CARTESIAN_POINT('Ctrl Pts',(-0.850258932191534,1.3,-0.527308329855003));
#8715=CARTESIAN_POINT('Ctrl Pts',(-0.881791875377343,1.3,-0.472691670144998));
#8716=CARTESIAN_POINT('Ctrl Pts',(-0.897143218189782,1.30632915724249,-0.442820664919227));
#8717=CARTESIAN_POINT('Ctrl Pts',(-0.92278792026947,1.33188468517318,-0.386546956384144));
#8718=CARTESIAN_POINT('Ctrl Pts',(-0.933155485613026,1.35110381617461,-0.360174810895352));
#8719=CARTESIAN_POINT('Ctrl Pts',(-0.948394987258249,1.39534588636318,-0.31788699900678));
#8720=CARTESIAN_POINT('Ctrl Pts',(-0.954308486908894,1.42336732874239,-0.299111603474268));
#8721=CARTESIAN_POINT('Ctrl Pts',(-0.961833761492986,1.48491957299737,-0.273949373987484));
#8722=CARTESIAN_POINT('Ctrl Pts',(-0.963525491562421,1.5184626473304,-0.267616567329818));
#8723=CARTESIAN_POINT('Ctrl Pts',(-0.963525491562421,1.5815373526696,-0.267616567329818));
#8724=CARTESIAN_POINT('Ctrl Pts',(-0.961833761492986,1.61508042700263,-0.273949373987484));
#8725=CARTESIAN_POINT('Ctrl Pts',(-0.954308486908894,1.67663267125761,-0.299111603474268));
#8726=CARTESIAN_POINT('Ctrl Pts',(-0.948394987258249,1.70465411363682,-0.31788699900678));
#8727=CARTESIAN_POINT('Ctrl Pts',(-0.933155485613026,1.74889618382539,-0.360174810895352));
#8728=CARTESIAN_POINT('Ctrl Pts',(-0.92278792026947,1.76811531482682,-0.386546956384144));
#8729=CARTESIAN_POINT('Ctrl Pts',(-0.897143218189782,1.79367084275751,-0.442820664919227));
#8730=CARTESIAN_POINT('Ctrl Pts',(-0.881791875377343,1.8,-0.472691670144998));
#8731=CARTESIAN_POINT('Ctrl Pts',(-0.850258932191534,1.8,-0.527308329855003));
#8732=CARTESIAN_POINT('Ctrl Pts',(-0.832065554235658,1.79367084275751,-0.555538485325664));
#8733=CARTESIAN_POINT('Ctrl Pts',(-0.796153444118959,1.76811531482682,-0.605884303066698));
#8734=CARTESIAN_POINT('Ctrl Pts',(-0.778498278845144,1.74889618382539,-0.62804895077401));
#8735=CARTESIAN_POINT('Ctrl Pts',(-0.749495710301794,1.70465411363682,-0.662390652284073));
#8736=CARTESIAN_POINT('Ctrl Pts',(-0.73619249062986,1.67663267125761,-0.676899590973058));
#8737=CARTESIAN_POINT('Ctrl Pts',(-0.718163997970498,1.61508042700263,-0.695997784676728));
#8738=CARTESIAN_POINT('Ctrl Pts',(-0.713525491562421,1.5815373526696,-0.700629269222037));
#8739=CARTESIAN_POINT('Ctrl Pts',(-0.713525491562421,1.55,-0.700629269222037));
#8740=CARTESIAN_POINT('',(-1.28744468918255,1.55,-1.03198167246111));
#8741=CARTESIAN_POINT('',(0.125,1.55,-0.21650635094611));
#8742=CARTESIAN_POINT('',(-1.42894191624432,1.3,-0.825000000000001));
#8743=CARTESIAN_POINT('Ctrl Pts',(-1.42894191624432,1.3,-0.825000000000001));
#8744=CARTESIAN_POINT('Ctrl Pts',(-1.4132207435299,1.3,-0.852229869895949));
#8745=CARTESIAN_POINT('Ctrl Pts',(-1.39561049050871,1.30629366210296,-0.880751161609749));
#8746=CARTESIAN_POINT('Ctrl Pts',(-1.36172049302549,1.33182222741682,-0.932292094146256));
#8747=CARTESIAN_POINT('Ctrl Pts',(-1.34548213209931,1.35105447038507,-0.955340251466735));
#8748=CARTESIAN_POINT('Ctrl Pts',(-1.31917543061769,1.39539254159618,-0.991349264982991));
#8749=CARTESIAN_POINT('Ctrl Pts',(-1.30734972067592,1.42347183818157,-1.00672880483252));
#8750=CARTESIAN_POINT('Ctrl Pts',(-1.29146042158868,1.48505200040818,-1.02703269653942));
#8751=CARTESIAN_POINT('Ctrl Pts',(-1.28744468918255,1.51855708359447,-1.03198167246111));
#8752=CARTESIAN_POINT('Ctrl Pts',(-1.28744468918255,1.55,-1.03198167246111));
#8753=CARTESIAN_POINT('',(-1.42894191624432,1.8,-0.825000000000001));
#8754=CARTESIAN_POINT('Ctrl Pts',(-1.42894191624432,1.8,-0.825000000000001));
#8755=CARTESIAN_POINT('Ctrl Pts',(-1.44466308895875,1.8,-0.797770130104052));
#8756=CARTESIAN_POINT('Ctrl Pts',(-1.46055812562105,1.79370633789704,-0.768258557763732));
#8757=CARTESIAN_POINT('Ctrl Pts',(-1.48824888379079,1.76817777258318,-0.713138492740816));
#8758=CARTESIAN_POINT('Ctrl Pts',(-1.50008999307766,1.74894552961493,-0.687551581002689));
#8759=CARTESIAN_POINT('Ctrl Pts',(-1.51812136280714,1.70460745840382,-0.646764802471699));
#8760=CARTESIAN_POINT('Ctrl Pts',(-1.52552758004446,1.67652816181843,-0.628833667319578));
#8761=CARTESIAN_POINT('Ctrl Pts',(-1.53516661651472,1.61494799959182,-0.60492118480825));
#8762=CARTESIAN_POINT('Ctrl Pts',(-1.53744468918255,1.58144291640553,-0.598968970568896));
#8763=CARTESIAN_POINT('Ctrl Pts',(-1.53744468918255,1.51855708359447,-0.598968970568896));
#8764=CARTESIAN_POINT('Ctrl Pts',(-1.53516661651472,1.48505200040818,-0.60492118480825));
#8765=CARTESIAN_POINT('Ctrl Pts',(-1.52552758004446,1.42347183818157,-0.628833667319578));
#8766=CARTESIAN_POINT('Ctrl Pts',(-1.51812136280714,1.39539254159618,-0.646764802471699));
#8767=CARTESIAN_POINT('Ctrl Pts',(-1.50008999307766,1.35105447038507,-0.687551581002689));
#8768=CARTESIAN_POINT('Ctrl Pts',(-1.48824888379079,1.33182222741682,-0.713138492740816));
#8769=CARTESIAN_POINT('Ctrl Pts',(-1.46055812562105,1.30629366210296,-0.768258557763732));
#8770=CARTESIAN_POINT('Ctrl Pts',(-1.44466308895875,1.3,-0.797770130104052));
#8771=CARTESIAN_POINT('Ctrl Pts',(-1.42894191624432,1.3,-0.825000000000001));
#8772=CARTESIAN_POINT('Ctrl Pts',(-1.28744468918255,1.55,-1.03198167246111));
#8773=CARTESIAN_POINT('Ctrl Pts',(-1.28744468918255,1.58144291640553,-1.03198167246111));
#8774=CARTESIAN_POINT('Ctrl Pts',(-1.29146042158868,1.61494799959182,-1.02703269653942));
#8775=CARTESIAN_POINT('Ctrl Pts',(-1.30734972067592,1.67652816181843,-1.00672880483252));
#8776=CARTESIAN_POINT('Ctrl Pts',(-1.31917543061769,1.70460745840382,-0.991349264982991));
#8777=CARTESIAN_POINT('Ctrl Pts',(-1.34548213209931,1.74894552961493,-0.955340251466734));
#8778=CARTESIAN_POINT('Ctrl Pts',(-1.36172049302549,1.76817777258318,-0.932292094146256));
#8779=CARTESIAN_POINT('Ctrl Pts',(-1.39561049050871,1.79370633789704,-0.880751161609749));
#8780=CARTESIAN_POINT('Ctrl Pts',(-1.4132207435299,1.8,-0.852229869895949));
#8781=CARTESIAN_POINT('Ctrl Pts',(-1.42894191624432,1.8,-0.825000000000001));
#8782=CARTESIAN_POINT('Origin',(0.,1.55,0.));
#8783=CARTESIAN_POINT('',(-1.65,0.85,-2.02066721859313E-16));
#8784=CARTESIAN_POINT('Origin',(0.,0.85,0.));
#8785=CARTESIAN_POINT('',(-1.65,2.25,-2.02066721859313E-16));
#8786=CARTESIAN_POINT('',(-1.65,1.55,-2.02066721859313E-16));
#8787=CARTESIAN_POINT('Origin',(0.,2.25,0.));
#8788=CARTESIAN_POINT('',(-1.42894191624432,1.3,0.825));
#8789=CARTESIAN_POINT('',(-1.42894191624432,1.8,0.825));
#8790=CARTESIAN_POINT('Ctrl Pts',(-1.42894191624432,1.3,0.825));
#8791=CARTESIAN_POINT('Ctrl Pts',(-1.44466308895875,1.3,0.797770130104051));
#8792=CARTESIAN_POINT('Ctrl Pts',(-1.46055812562105,1.30629366210296,0.768258557763731));
#8793=CARTESIAN_POINT('Ctrl Pts',(-1.48824888379079,1.33182222741682,0.713138492740815));
#8794=CARTESIAN_POINT('Ctrl Pts',(-1.50008999307766,1.35105447038507,0.687551581002688));
#8795=CARTESIAN_POINT('Ctrl Pts',(-1.51812136280714,1.39539254159618,0.646764802471698));
#8796=CARTESIAN_POINT('Ctrl Pts',(-1.52552758004446,1.42347183818157,0.628833667319577));
#8797=CARTESIAN_POINT('Ctrl Pts',(-1.53516661651472,1.48505200040818,0.604921184808249));
#8798=CARTESIAN_POINT('Ctrl Pts',(-1.53744468918255,1.51855708359447,0.598968970568895));
#8799=CARTESIAN_POINT('Ctrl Pts',(-1.53744468918255,1.58144291640553,0.598968970568895));
#8800=CARTESIAN_POINT('Ctrl Pts',(-1.53516661651472,1.61494799959182,0.604921184808249));
#8801=CARTESIAN_POINT('Ctrl Pts',(-1.52552758004446,1.67652816181843,0.628833667319577));
#8802=CARTESIAN_POINT('Ctrl Pts',(-1.51812136280714,1.70460745840382,0.646764802471698));
#8803=CARTESIAN_POINT('Ctrl Pts',(-1.50008999307766,1.74894552961493,0.687551581002688));
#8804=CARTESIAN_POINT('Ctrl Pts',(-1.48824888379079,1.76817777258318,0.713138492740815));
#8805=CARTESIAN_POINT('Ctrl Pts',(-1.46055812562105,1.79370633789704,0.768258557763731));
#8806=CARTESIAN_POINT('Ctrl Pts',(-1.44466308895875,1.8,0.797770130104051));
#8807=CARTESIAN_POINT('Ctrl Pts',(-1.42894191624432,1.8,0.825));
#8808=CARTESIAN_POINT('',(-1.28744468918255,1.55,1.03198167246111));
#8809=CARTESIAN_POINT('Ctrl Pts',(-1.42894191624432,1.8,0.825));
#8810=CARTESIAN_POINT('Ctrl Pts',(-1.4132207435299,1.8,0.852229869895948));
#8811=CARTESIAN_POINT('Ctrl Pts',(-1.39561049050871,1.79370633789704,0.880751161609747));
#8812=CARTESIAN_POINT('Ctrl Pts',(-1.36172049302549,1.76817777258318,0.932292094146255));
#8813=CARTESIAN_POINT('Ctrl Pts',(-1.34548213209931,1.74894552961493,0.955340251466733));
#8814=CARTESIAN_POINT('Ctrl Pts',(-1.31917543061769,1.70460745840382,0.991349264982989));
#8815=CARTESIAN_POINT('Ctrl Pts',(-1.30734972067592,1.67652816181843,1.00672880483252));
#8816=CARTESIAN_POINT('Ctrl Pts',(-1.29146042158868,1.61494799959182,1.02703269653942));
#8817=CARTESIAN_POINT('Ctrl Pts',(-1.28744468918255,1.58144291640553,1.03198167246111));
#8818=CARTESIAN_POINT('Ctrl Pts',(-1.28744468918255,1.55,1.03198167246111));
#8819=CARTESIAN_POINT('Ctrl Pts',(-1.28744468918255,1.55,1.03198167246111));
#8820=CARTESIAN_POINT('Ctrl Pts',(-1.28744468918255,1.51855708359447,1.03198167246111));
#8821=CARTESIAN_POINT('Ctrl Pts',(-1.29146042158868,1.48505200040818,1.02703269653942));
#8822=CARTESIAN_POINT('Ctrl Pts',(-1.30734972067592,1.42347183818157,1.00672880483252));
#8823=CARTESIAN_POINT('Ctrl Pts',(-1.31917543061769,1.39539254159618,0.99134926498299));
#8824=CARTESIAN_POINT('Ctrl Pts',(-1.34548213209931,1.35105447038508,0.955340251466733));
#8825=CARTESIAN_POINT('Ctrl Pts',(-1.36172049302549,1.33182222741682,0.932292094146255));
#8826=CARTESIAN_POINT('Ctrl Pts',(-1.39561049050871,1.30629366210296,0.880751161609748));
#8827=CARTESIAN_POINT('Ctrl Pts',(-1.4132207435299,1.3,0.852229869895949));
#8828=CARTESIAN_POINT('Ctrl Pts',(-1.42894191624432,1.3,0.825));
#8829=CARTESIAN_POINT('',(1.42894191624432,1.8,-0.825));
#8830=CARTESIAN_POINT('',(1.42894191624432,1.3,-0.825));
#8831=CARTESIAN_POINT('Ctrl Pts',(1.42894191624432,1.8,-0.825));
#8832=CARTESIAN_POINT('Ctrl Pts',(1.4132207435299,1.8,-0.852229869895949));
#8833=CARTESIAN_POINT('Ctrl Pts',(1.39561049050871,1.79370633789704,-0.880751161609748));
#8834=CARTESIAN_POINT('Ctrl Pts',(1.36172049302549,1.76817777258318,-0.932292094146255));
#8835=CARTESIAN_POINT('Ctrl Pts',(1.34548213209931,1.74894552961493,-0.955340251466734));
#8836=CARTESIAN_POINT('Ctrl Pts',(1.31917543061769,1.70460745840382,-0.99134926498299));
#8837=CARTESIAN_POINT('Ctrl Pts',(1.30734972067592,1.67652816181843,-1.00672880483252));
#8838=CARTESIAN_POINT('Ctrl Pts',(1.29146042158868,1.61494799959182,-1.02703269653942));
#8839=CARTESIAN_POINT('Ctrl Pts',(1.28744468918255,1.58144291640553,-1.03198167246111));
#8840=CARTESIAN_POINT('Ctrl Pts',(1.28744468918255,1.51855708359447,-1.03198167246111));
#8841=CARTESIAN_POINT('Ctrl Pts',(1.29146042158868,1.48505200040818,-1.02703269653942));
#8842=CARTESIAN_POINT('Ctrl Pts',(1.30734972067592,1.42347183818157,-1.00672880483252));
#8843=CARTESIAN_POINT('Ctrl Pts',(1.31917543061769,1.39539254159618,-0.99134926498299));
#8844=CARTESIAN_POINT('Ctrl Pts',(1.34548213209931,1.35105447038507,-0.955340251466734));
#8845=CARTESIAN_POINT('Ctrl Pts',(1.36172049302549,1.33182222741682,-0.932292094146255));
#8846=CARTESIAN_POINT('Ctrl Pts',(1.39561049050871,1.30629366210296,-0.880751161609748));
#8847=CARTESIAN_POINT('Ctrl Pts',(1.4132207435299,1.3,-0.852229869895948));
#8848=CARTESIAN_POINT('Ctrl Pts',(1.42894191624432,1.3,-0.825));
#8849=CARTESIAN_POINT('',(1.53744468918255,1.55,-0.598968970568895));
#8850=CARTESIAN_POINT('Ctrl Pts',(1.42894191624432,1.3,-0.825));
#8851=CARTESIAN_POINT('Ctrl Pts',(1.44466308895875,1.3,-0.797770130104051));
#8852=CARTESIAN_POINT('Ctrl Pts',(1.46055812562105,1.30629366210296,-0.768258557763731));
#8853=CARTESIAN_POINT('Ctrl Pts',(1.48824888379079,1.33182222741682,-0.713138492740815));
#8854=CARTESIAN_POINT('Ctrl Pts',(1.50008999307766,1.35105447038507,-0.687551581002688));
#8855=CARTESIAN_POINT('Ctrl Pts',(1.51812136280714,1.39539254159618,-0.646764802471698));
#8856=CARTESIAN_POINT('Ctrl Pts',(1.52552758004446,1.42347183818157,-0.628833667319577));
#8857=CARTESIAN_POINT('Ctrl Pts',(1.53516661651472,1.48505200040818,-0.604921184808249));
#8858=CARTESIAN_POINT('Ctrl Pts',(1.53744468918255,1.51855708359447,-0.598968970568895));
#8859=CARTESIAN_POINT('Ctrl Pts',(1.53744468918255,1.55,-0.598968970568895));
#8860=CARTESIAN_POINT('Ctrl Pts',(1.53744468918255,1.55,-0.598968970568895));
#8861=CARTESIAN_POINT('Ctrl Pts',(1.53744468918255,1.58144291640553,-0.598968970568895));
#8862=CARTESIAN_POINT('Ctrl Pts',(1.53516661651472,1.61494799959182,-0.604921184808249));
#8863=CARTESIAN_POINT('Ctrl Pts',(1.52552758004446,1.67652816181843,-0.628833667319577));
#8864=CARTESIAN_POINT('Ctrl Pts',(1.51812136280714,1.70460745840382,-0.646764802471698));
#8865=CARTESIAN_POINT('Ctrl Pts',(1.50008999307766,1.74894552961493,-0.687551581002688));
#8866=CARTESIAN_POINT('Ctrl Pts',(1.48824888379079,1.76817777258318,-0.713138492740815));
#8867=CARTESIAN_POINT('Ctrl Pts',(1.46055812562105,1.79370633789704,-0.768258557763731));
#8868=CARTESIAN_POINT('Ctrl Pts',(1.44466308895875,1.8,-0.797770130104051));
#8869=CARTESIAN_POINT('Ctrl Pts',(1.42894191624432,1.8,-0.825));
#8870=CARTESIAN_POINT('',(0.,1.3,-1.65));
#8871=CARTESIAN_POINT('',(0.,1.8,-1.65));
#8872=CARTESIAN_POINT('Ctrl Pts',(1.38777878078145E-17,1.3,-1.65));
#8873=CARTESIAN_POINT('Ctrl Pts',(0.0314423454288489,1.3,-1.65));
#8874=CARTESIAN_POINT('Ctrl Pts',(0.0649476351123396,1.30629366210296,-1.64900971937348));
#8875=CARTESIAN_POINT('Ctrl Pts',(0.126528390765307,1.33182222741682,-1.64543058688707));
#8876=CARTESIAN_POINT('Ctrl Pts',(0.154607860978348,1.35105447038507,-1.64289183246942));
#8877=CARTESIAN_POINT('Ctrl Pts',(0.198945932189457,1.39539254159618,-1.63811406745469));
#8878=CARTESIAN_POINT('Ctrl Pts',(0.218177859368546,1.42347183818157,-1.63556247215209));
#8879=CARTESIAN_POINT('Ctrl Pts',(0.243706194926033,1.48505200040818,-1.63195388134767));
#8880=CARTESIAN_POINT('Ctrl Pts',(0.25,1.51855708359447,-1.63095064303001));
#8881=CARTESIAN_POINT('Ctrl Pts',(0.25,1.58144291640553,-1.63095064303001));
#8882=CARTESIAN_POINT('Ctrl Pts',(0.243706194926033,1.61494799959182,-1.63195388134767));
#8883=CARTESIAN_POINT('Ctrl Pts',(0.218177859368546,1.67652816181843,-1.63556247215209));
#8884=CARTESIAN_POINT('Ctrl Pts',(0.198945932189457,1.70460745840382,-1.63811406745469));
#8885=CARTESIAN_POINT('Ctrl Pts',(0.154607860978349,1.74894552961493,-1.64289183246942));
#8886=CARTESIAN_POINT('Ctrl Pts',(0.126528390765307,1.76817777258318,-1.64543058688707));
#8887=CARTESIAN_POINT('Ctrl Pts',(0.0649476351123398,1.79370633789704,-1.64900971937348));
#8888=CARTESIAN_POINT('Ctrl Pts',(0.031442345428849,1.8,-1.65));
#8889=CARTESIAN_POINT('Ctrl Pts',(7.63278329429795E-17,1.8,-1.65));
#8890=CARTESIAN_POINT('',(-0.25,1.55,-1.63095064303001));
#8891=CARTESIAN_POINT('Ctrl Pts',(9.0205620750794E-17,1.8,-1.65));
#8892=CARTESIAN_POINT('Ctrl Pts',(-0.0314423454288488,1.8,-1.65));
#8893=CARTESIAN_POINT('Ctrl Pts',(-0.0649476351123396,1.79370633789704,
-1.64900971937348));
#8894=CARTESIAN_POINT('Ctrl Pts',(-0.126528390765307,1.76817777258318,-1.64543058688707));
#8895=CARTESIAN_POINT('Ctrl Pts',(-0.154607860978348,1.74894552961493,-1.64289183246942));
#8896=CARTESIAN_POINT('Ctrl Pts',(-0.198945932189456,1.70460745840382,-1.63811406745469));
#8897=CARTESIAN_POINT('Ctrl Pts',(-0.218177859368546,1.67652816181843,-1.63556247215209));
#8898=CARTESIAN_POINT('Ctrl Pts',(-0.243706194926033,1.61494799959182,-1.63195388134767));
#8899=CARTESIAN_POINT('Ctrl Pts',(-0.25,1.58144291640553,-1.63095064303001));
#8900=CARTESIAN_POINT('Ctrl Pts',(-0.25,1.55,-1.63095064303001));
#8901=CARTESIAN_POINT('Ctrl Pts',(-0.25,1.55,-1.63095064303001));
#8902=CARTESIAN_POINT('Ctrl Pts',(-0.25,1.51855708359447,-1.63095064303001));
#8903=CARTESIAN_POINT('Ctrl Pts',(-0.243706194926033,1.48505200040818,-1.63195388134767));
#8904=CARTESIAN_POINT('Ctrl Pts',(-0.218177859368546,1.42347183818157,-1.63556247215209));
#8905=CARTESIAN_POINT('Ctrl Pts',(-0.198945932189457,1.39539254159618,-1.63811406745469));
#8906=CARTESIAN_POINT('Ctrl Pts',(-0.154607860978349,1.35105447038507,-1.64289183246942));
#8907=CARTESIAN_POINT('Ctrl Pts',(-0.126528390765307,1.33182222741682,-1.64543058688707));
#8908=CARTESIAN_POINT('Ctrl Pts',(-0.0649476351123398,1.30629366210296,
-1.64900971937348));
#8909=CARTESIAN_POINT('Ctrl Pts',(-0.031442345428849,1.3,-1.65));
#8910=CARTESIAN_POINT('Ctrl Pts',(-4.85722573273506E-17,1.3,-1.65));
#8911=CARTESIAN_POINT('',(0.,1.8,1.65));
#8912=CARTESIAN_POINT('',(0.,1.3,1.65));
#8913=CARTESIAN_POINT('Ctrl Pts',(8.32667268468867E-17,1.8,1.65));
#8914=CARTESIAN_POINT('Ctrl Pts',(0.031442345428849,1.8,1.65));
#8915=CARTESIAN_POINT('Ctrl Pts',(0.0649476351123398,1.79370633789704,1.64900971937348));
#8916=CARTESIAN_POINT('Ctrl Pts',(0.126528390765307,1.76817777258318,1.64543058688707));
#8917=CARTESIAN_POINT('Ctrl Pts',(0.154607860978349,1.74894552961493,1.64289183246942));
#8918=CARTESIAN_POINT('Ctrl Pts',(0.198945932189457,1.70460745840382,1.63811406745469));
#8919=CARTESIAN_POINT('Ctrl Pts',(0.218177859368546,1.67652816181843,1.63556247215209));
#8920=CARTESIAN_POINT('Ctrl Pts',(0.243706194926033,1.61494799959182,1.63195388134767));
#8921=CARTESIAN_POINT('Ctrl Pts',(0.25,1.58144291640553,1.63095064303001));
#8922=CARTESIAN_POINT('Ctrl Pts',(0.25,1.51855708359447,1.63095064303001));
#8923=CARTESIAN_POINT('Ctrl Pts',(0.243706194926033,1.48505200040818,1.63195388134767));
#8924=CARTESIAN_POINT('Ctrl Pts',(0.218177859368546,1.42347183818157,1.63556247215209));
#8925=CARTESIAN_POINT('Ctrl Pts',(0.198945932189457,1.39539254159618,1.63811406745469));
#8926=CARTESIAN_POINT('Ctrl Pts',(0.154607860978348,1.35105447038507,1.64289183246942));
#8927=CARTESIAN_POINT('Ctrl Pts',(0.126528390765307,1.33182222741682,1.64543058688707));
#8928=CARTESIAN_POINT('Ctrl Pts',(0.0649476351123397,1.30629366210296,1.64900971937348));
#8929=CARTESIAN_POINT('Ctrl Pts',(0.0314423454288488,1.3,1.65));
#8930=CARTESIAN_POINT('Ctrl Pts',(-1.38777878078145E-17,1.3,1.65));
#8931=CARTESIAN_POINT('',(-0.25,1.55,1.63095064303001));
#8932=CARTESIAN_POINT('Ctrl Pts',(-5.55111512312578E-17,1.3,1.65));
#8933=CARTESIAN_POINT('Ctrl Pts',(-0.031442345428849,1.3,1.65));
#8934=CARTESIAN_POINT('Ctrl Pts',(-0.0649476351123398,1.30629366210296,
1.64900971937348));
#8935=CARTESIAN_POINT('Ctrl Pts',(-0.126528390765307,1.33182222741682,1.64543058688707));
#8936=CARTESIAN_POINT('Ctrl Pts',(-0.154607860978349,1.35105447038507,1.64289183246942));
#8937=CARTESIAN_POINT('Ctrl Pts',(-0.198945932189457,1.39539254159618,1.63811406745469));
#8938=CARTESIAN_POINT('Ctrl Pts',(-0.218177859368546,1.42347183818157,1.63556247215209));
#8939=CARTESIAN_POINT('Ctrl Pts',(-0.243706194926033,1.48505200040818,1.63195388134767));
#8940=CARTESIAN_POINT('Ctrl Pts',(-0.25,1.51855708359447,1.63095064303001));
#8941=CARTESIAN_POINT('Ctrl Pts',(-0.25,1.55,1.63095064303001));
#8942=CARTESIAN_POINT('Ctrl Pts',(-0.25,1.55,1.63095064303001));
#8943=CARTESIAN_POINT('Ctrl Pts',(-0.25,1.58144291640553,1.63095064303001));
#8944=CARTESIAN_POINT('Ctrl Pts',(-0.243706194926033,1.61494799959182,1.63195388134767));
#8945=CARTESIAN_POINT('Ctrl Pts',(-0.218177859368546,1.67652816181843,1.63556247215209));
#8946=CARTESIAN_POINT('Ctrl Pts',(-0.198945932189456,1.70460745840382,1.63811406745469));
#8947=CARTESIAN_POINT('Ctrl Pts',(-0.154607860978348,1.74894552961493,1.64289183246942));
#8948=CARTESIAN_POINT('Ctrl Pts',(-0.126528390765307,1.76817777258318,1.64543058688707));
#8949=CARTESIAN_POINT('Ctrl Pts',(-0.0649476351123396,1.79370633789704,
1.64900971937348));
#8950=CARTESIAN_POINT('Ctrl Pts',(-0.0314423454288488,1.8,1.65));
#8951=CARTESIAN_POINT('Ctrl Pts',(7.63278329429795E-17,1.8,1.65));
#8952=CARTESIAN_POINT('Origin',(0.,1.55,0.));
#8953=CARTESIAN_POINT('',(-0.713525491562421,1.55,0.700629269222037));
#8954=CARTESIAN_POINT('',(0.125,1.55,0.21650635094611));
#8955=CARTESIAN_POINT('Ctrl Pts',(-0.713525491562421,1.55,0.700629269222037));
#8956=CARTESIAN_POINT('Ctrl Pts',(-0.713525491562421,1.5815373526696,0.700629269222037));
#8957=CARTESIAN_POINT('Ctrl Pts',(-0.718163997970498,1.61508042700263,0.695997784676727));
#8958=CARTESIAN_POINT('Ctrl Pts',(-0.73619249062986,1.67663267125761,0.676899590973058));
#8959=CARTESIAN_POINT('Ctrl Pts',(-0.749495710301795,1.70465411363682,0.662390652284073));
#8960=CARTESIAN_POINT('Ctrl Pts',(-0.778498278845144,1.74889618382539,0.628048950774009));
#8961=CARTESIAN_POINT('Ctrl Pts',(-0.796153444118959,1.76811531482682,0.605884303066698));
#8962=CARTESIAN_POINT('Ctrl Pts',(-0.832065554235658,1.79367084275751,0.555538485325663));
#8963=CARTESIAN_POINT('Ctrl Pts',(-0.850258932191534,1.8,0.527308329855002));
#8964=CARTESIAN_POINT('Ctrl Pts',(-0.881791875377343,1.8,0.472691670144998));
#8965=CARTESIAN_POINT('Ctrl Pts',(-0.897143218189782,1.79367084275751,0.442820664919227));
#8966=CARTESIAN_POINT('Ctrl Pts',(-0.92278792026947,1.76811531482682,0.386546956384144));
#8967=CARTESIAN_POINT('Ctrl Pts',(-0.933155485613026,1.74889618382539,0.360174810895352));
#8968=CARTESIAN_POINT('Ctrl Pts',(-0.948394987258249,1.70465411363682,0.31788699900678));
#8969=CARTESIAN_POINT('Ctrl Pts',(-0.954308486908894,1.67663267125761,0.299111603474267));
#8970=CARTESIAN_POINT('Ctrl Pts',(-0.961833761492987,1.61508042700263,0.273949373987484));
#8971=CARTESIAN_POINT('Ctrl Pts',(-0.963525491562421,1.5815373526696,0.267616567329817));
#8972=CARTESIAN_POINT('Ctrl Pts',(-0.963525491562421,1.5184626473304,0.267616567329817));
#8973=CARTESIAN_POINT('Ctrl Pts',(-0.961833761492987,1.48491957299737,0.273949373987484));
#8974=CARTESIAN_POINT('Ctrl Pts',(-0.954308486908894,1.42336732874239,0.299111603474267));
#8975=CARTESIAN_POINT('Ctrl Pts',(-0.948394987258249,1.39534588636318,0.31788699900678));
#8976=CARTESIAN_POINT('Ctrl Pts',(-0.933155485613026,1.35110381617461,0.360174810895352));
#8977=CARTESIAN_POINT('Ctrl Pts',(-0.92278792026947,1.33188468517318,0.386546956384144));
#8978=CARTESIAN_POINT('Ctrl Pts',(-0.897143218189782,1.30632915724249,0.442820664919227));
#8979=CARTESIAN_POINT('Ctrl Pts',(-0.881791875377343,1.3,0.472691670144998));
#8980=CARTESIAN_POINT('Ctrl Pts',(-0.850258932191534,1.3,0.527308329855002));
#8981=CARTESIAN_POINT('Ctrl Pts',(-0.832065554235658,1.30632915724249,0.555538485325663));
#8982=CARTESIAN_POINT('Ctrl Pts',(-0.796153444118959,1.33188468517318,0.605884303066698));
#8983=CARTESIAN_POINT('Ctrl Pts',(-0.778498278845144,1.35110381617461,0.628048950774009));
#8984=CARTESIAN_POINT('Ctrl Pts',(-0.749495710301795,1.39534588636318,0.662390652284073));
#8985=CARTESIAN_POINT('Ctrl Pts',(-0.73619249062986,1.42336732874239,0.676899590973058));
#8986=CARTESIAN_POINT('Ctrl Pts',(-0.718163997970498,1.48491957299737,0.695997784676727));
#8987=CARTESIAN_POINT('Ctrl Pts',(-0.713525491562421,1.5184626473304,0.700629269222037));
#8988=CARTESIAN_POINT('Ctrl Pts',(-0.713525491562421,1.55,0.700629269222037));
#8989=CARTESIAN_POINT('Origin',(0.,1.55,0.));
#8990=CARTESIAN_POINT('',(0.963525491562421,1.55,-0.267616567329817));
#8991=CARTESIAN_POINT('Ctrl Pts',(0.963525491562421,1.55,-0.267616567329817));
#8992=CARTESIAN_POINT('Ctrl Pts',(0.963525491562421,1.5184626473304,-0.267616567329817));
#8993=CARTESIAN_POINT('Ctrl Pts',(0.961833761492987,1.48491957299737,-0.273949373987484));
#8994=CARTESIAN_POINT('Ctrl Pts',(0.954308486908894,1.42336732874239,-0.299111603474267));
#8995=CARTESIAN_POINT('Ctrl Pts',(0.948394987258249,1.39534588636318,-0.31788699900678));
#8996=CARTESIAN_POINT('Ctrl Pts',(0.933155485613026,1.35110381617461,-0.360174810895352));
#8997=CARTESIAN_POINT('Ctrl Pts',(0.92278792026947,1.33188468517318,-0.386546956384144));
#8998=CARTESIAN_POINT('Ctrl Pts',(0.897143218189782,1.30632915724249,-0.442820664919227));
#8999=CARTESIAN_POINT('Ctrl Pts',(0.881791875377343,1.3,-0.472691670144998));
#9000=CARTESIAN_POINT('Ctrl Pts',(0.850258932191534,1.3,-0.527308329855002));
#9001=CARTESIAN_POINT('Ctrl Pts',(0.832065554235658,1.30632915724249,-0.555538485325663));
#9002=CARTESIAN_POINT('Ctrl Pts',(0.796153444118959,1.33188468517318,-0.605884303066698));
#9003=CARTESIAN_POINT('Ctrl Pts',(0.778498278845144,1.35110381617461,-0.628048950774009));
#9004=CARTESIAN_POINT('Ctrl Pts',(0.749495710301795,1.39534588636318,-0.662390652284073));
#9005=CARTESIAN_POINT('Ctrl Pts',(0.73619249062986,1.42336732874239,-0.676899590973058));
#9006=CARTESIAN_POINT('Ctrl Pts',(0.718163997970498,1.48491957299737,-0.695997784676727));
#9007=CARTESIAN_POINT('Ctrl Pts',(0.713525491562421,1.5184626473304,-0.700629269222037));
#9008=CARTESIAN_POINT('Ctrl Pts',(0.713525491562421,1.5815373526696,-0.700629269222037));
#9009=CARTESIAN_POINT('Ctrl Pts',(0.718163997970498,1.61508042700263,-0.695997784676727));
#9010=CARTESIAN_POINT('Ctrl Pts',(0.73619249062986,1.67663267125761,-0.676899590973058));
#9011=CARTESIAN_POINT('Ctrl Pts',(0.749495710301795,1.70465411363682,-0.662390652284073));
#9012=CARTESIAN_POINT('Ctrl Pts',(0.778498278845144,1.74889618382539,-0.628048950774009));
#9013=CARTESIAN_POINT('Ctrl Pts',(0.796153444118959,1.76811531482682,-0.605884303066698));
#9014=CARTESIAN_POINT('Ctrl Pts',(0.832065554235658,1.79367084275751,-0.555538485325663));
#9015=CARTESIAN_POINT('Ctrl Pts',(0.850258932191534,1.8,-0.527308329855002));
#9016=CARTESIAN_POINT('Ctrl Pts',(0.881791875377343,1.8,-0.472691670144998));
#9017=CARTESIAN_POINT('Ctrl Pts',(0.897143218189782,1.79367084275751,-0.442820664919227));
#9018=CARTESIAN_POINT('Ctrl Pts',(0.92278792026947,1.76811531482682,-0.386546956384144));
#9019=CARTESIAN_POINT('Ctrl Pts',(0.933155485613026,1.74889618382539,-0.360174810895352));
#9020=CARTESIAN_POINT('Ctrl Pts',(0.948394987258249,1.70465411363682,-0.31788699900678));
#9021=CARTESIAN_POINT('Ctrl Pts',(0.954308486908894,1.67663267125761,-0.299111603474267));
#9022=CARTESIAN_POINT('Ctrl Pts',(0.961833761492987,1.61508042700263,-0.273949373987484));
#9023=CARTESIAN_POINT('Ctrl Pts',(0.963525491562421,1.5815373526696,-0.267616567329817));
#9024=CARTESIAN_POINT('Ctrl Pts',(0.963525491562421,1.55,-0.267616567329817));
#9025=CARTESIAN_POINT('',(0.125,1.55,0.21650635094611));
#9026=CARTESIAN_POINT('Origin',(0.,1.55,0.));
#9027=CARTESIAN_POINT('',(-0.25,1.55,-0.968245836551854));
#9028=CARTESIAN_POINT('',(-0.25,1.55,0.));
#9029=CARTESIAN_POINT('Ctrl Pts',(-0.25,1.55,-0.968245836551854));
#9030=CARTESIAN_POINT('Ctrl Pts',(-0.25,1.5815373526696,-0.968245836551854));
#9031=CARTESIAN_POINT('Ctrl Pts',(-0.243669763522489,1.61508042700263,-0.969947158664211));
#9032=CARTESIAN_POINT('Ctrl Pts',(-0.218115996279034,1.67663267125761,-0.976011194447325));
#9033=CARTESIAN_POINT('Ctrl Pts',(-0.198899276956455,1.70465411363682,-0.980277651290853));
#9034=CARTESIAN_POINT('Ctrl Pts',(-0.154657206767882,1.74889618382539,-0.988223761669361));
#9035=CARTESIAN_POINT('Ctrl Pts',(-0.126634476150511,1.76811531482682,-0.992431259450842));
#9036=CARTESIAN_POINT('Ctrl Pts',(-0.0650776639541238,1.79367084275751,
-0.99835915024489));
#9037=CARTESIAN_POINT('Ctrl Pts',(-0.0315329431858092,1.8,-1.));
#9038=CARTESIAN_POINT('Ctrl Pts',(0.0315329431858092,1.8,-1.));
#9039=CARTESIAN_POINT('Ctrl Pts',(0.0650776639541238,1.79367084275751,-0.99835915024489));
#9040=CARTESIAN_POINT('Ctrl Pts',(0.126634476150511,1.76811531482682,-0.992431259450842));
#9041=CARTESIAN_POINT('Ctrl Pts',(0.154657206767882,1.74889618382539,-0.988223761669361));
#9042=CARTESIAN_POINT('Ctrl Pts',(0.198899276956455,1.70465411363682,-0.980277651290853));
#9043=CARTESIAN_POINT('Ctrl Pts',(0.218115996279034,1.67663267125761,-0.976011194447325));
#9044=CARTESIAN_POINT('Ctrl Pts',(0.243669763522488,1.61508042700263,-0.969947158664211));
#9045=CARTESIAN_POINT('Ctrl Pts',(0.25,1.5815373526696,-0.968245836551854));
#9046=CARTESIAN_POINT('Ctrl Pts',(0.25,1.5184626473304,-0.968245836551854));
#9047=CARTESIAN_POINT('Ctrl Pts',(0.243669763522488,1.48491957299737,-0.969947158664211));
#9048=CARTESIAN_POINT('Ctrl Pts',(0.218115996279034,1.42336732874239,-0.976011194447325));
#9049=CARTESIAN_POINT('Ctrl Pts',(0.198899276956455,1.39534588636318,-0.980277651290853));
#9050=CARTESIAN_POINT('Ctrl Pts',(0.154657206767882,1.35110381617461,-0.988223761669361));
#9051=CARTESIAN_POINT('Ctrl Pts',(0.126634476150511,1.33188468517318,-0.992431259450842));
#9052=CARTESIAN_POINT('Ctrl Pts',(0.0650776639541239,1.30632915724249,-0.99835915024489));
#9053=CARTESIAN_POINT('Ctrl Pts',(0.0315329431858092,1.3,-1.));
#9054=CARTESIAN_POINT('Ctrl Pts',(-0.0315329431858092,1.3,-1.));
#9055=CARTESIAN_POINT('Ctrl Pts',(-0.0650776639541239,1.30632915724249,
-0.99835915024489));
#9056=CARTESIAN_POINT('Ctrl Pts',(-0.126634476150511,1.33188468517318,-0.992431259450842));
#9057=CARTESIAN_POINT('Ctrl Pts',(-0.154657206767882,1.35110381617461,-0.988223761669361));
#9058=CARTESIAN_POINT('Ctrl Pts',(-0.198899276956455,1.39534588636318,-0.980277651290853));
#9059=CARTESIAN_POINT('Ctrl Pts',(-0.218115996279034,1.42336732874239,-0.976011194447325));
#9060=CARTESIAN_POINT('Ctrl Pts',(-0.243669763522489,1.48491957299737,-0.969947158664211));
#9061=CARTESIAN_POINT('Ctrl Pts',(-0.25,1.5184626473304,-0.968245836551854));
#9062=CARTESIAN_POINT('Ctrl Pts',(-0.25,1.55,-0.968245836551854));
#9063=CARTESIAN_POINT('Origin',(0.,1.55,0.));
#9064=CARTESIAN_POINT('',(-0.25,1.55,0.968245836551854));
#9065=CARTESIAN_POINT('Ctrl Pts',(-0.25,1.55,0.968245836551854));
#9066=CARTESIAN_POINT('Ctrl Pts',(-0.25,1.5184626473304,0.968245836551854));
#9067=CARTESIAN_POINT('Ctrl Pts',(-0.243669763522489,1.48491957299737,0.969947158664211));
#9068=CARTESIAN_POINT('Ctrl Pts',(-0.218115996279034,1.42336732874239,0.976011194447325));
#9069=CARTESIAN_POINT('Ctrl Pts',(-0.198899276956455,1.39534588636318,0.980277651290853));
#9070=CARTESIAN_POINT('Ctrl Pts',(-0.154657206767882,1.35110381617461,0.988223761669361));
#9071=CARTESIAN_POINT('Ctrl Pts',(-0.126634476150511,1.33188468517318,0.992431259450842));
#9072=CARTESIAN_POINT('Ctrl Pts',(-0.065077663954124,1.30632915724249,0.99835915024489));
#9073=CARTESIAN_POINT('Ctrl Pts',(-0.0315329431858092,1.3,1.));
#9074=CARTESIAN_POINT('Ctrl Pts',(0.0315329431858092,1.3,1.));
#9075=CARTESIAN_POINT('Ctrl Pts',(0.065077663954124,1.30632915724249,0.99835915024489));
#9076=CARTESIAN_POINT('Ctrl Pts',(0.126634476150511,1.33188468517318,0.992431259450842));
#9077=CARTESIAN_POINT('Ctrl Pts',(0.154657206767882,1.35110381617461,0.988223761669361));
#9078=CARTESIAN_POINT('Ctrl Pts',(0.198899276956455,1.39534588636318,0.980277651290853));
#9079=CARTESIAN_POINT('Ctrl Pts',(0.218115996279034,1.42336732874239,0.976011194447325));
#9080=CARTESIAN_POINT('Ctrl Pts',(0.243669763522488,1.48491957299737,0.969947158664211));
#9081=CARTESIAN_POINT('Ctrl Pts',(0.25,1.5184626473304,0.968245836551854));
#9082=CARTESIAN_POINT('Ctrl Pts',(0.25,1.5815373526696,0.968245836551854));
#9083=CARTESIAN_POINT('Ctrl Pts',(0.243669763522488,1.61508042700263,0.969947158664211));
#9084=CARTESIAN_POINT('Ctrl Pts',(0.218115996279034,1.67663267125761,0.976011194447325));
#9085=CARTESIAN_POINT('Ctrl Pts',(0.198899276956455,1.70465411363682,0.980277651290853));
#9086=CARTESIAN_POINT('Ctrl Pts',(0.154657206767882,1.74889618382539,0.988223761669361));
#9087=CARTESIAN_POINT('Ctrl Pts',(0.126634476150511,1.76811531482682,0.992431259450842));
#9088=CARTESIAN_POINT('Ctrl Pts',(0.0650776639541239,1.79367084275751,0.99835915024489));
#9089=CARTESIAN_POINT('Ctrl Pts',(0.0315329431858092,1.8,1.));
#9090=CARTESIAN_POINT('Ctrl Pts',(-0.0315329431858092,1.8,1.));
#9091=CARTESIAN_POINT('Ctrl Pts',(-0.0650776639541239,1.79367084275751,
0.99835915024489));
#9092=CARTESIAN_POINT('Ctrl Pts',(-0.126634476150511,1.76811531482682,0.992431259450842));
#9093=CARTESIAN_POINT('Ctrl Pts',(-0.154657206767882,1.74889618382539,0.988223761669361));
#9094=CARTESIAN_POINT('Ctrl Pts',(-0.198899276956455,1.70465411363682,0.980277651290853));
#9095=CARTESIAN_POINT('Ctrl Pts',(-0.218115996279034,1.67663267125761,0.976011194447325));
#9096=CARTESIAN_POINT('Ctrl Pts',(-0.243669763522489,1.61508042700263,0.969947158664211));
#9097=CARTESIAN_POINT('Ctrl Pts',(-0.25,1.5815373526696,0.968245836551854));
#9098=CARTESIAN_POINT('Ctrl Pts',(-0.25,1.55,0.968245836551854));
#9099=CARTESIAN_POINT('',(-0.25,1.55,0.));
#9100=CARTESIAN_POINT('Origin',(1.65,2.25,0.));
#9101=CARTESIAN_POINT('',(-1.,2.25,-1.22464679914735E-16));
#9102=CARTESIAN_POINT('Origin',(0.,2.25,0.));
#9103=CARTESIAN_POINT('Origin',(1.75,0.85,0.));
#9104=CARTESIAN_POINT('',(-1.75,0.85,-2.14313189850787E-16));
#9105=CARTESIAN_POINT('Origin',(0.,0.85,0.));
#9106=CARTESIAN_POINT('Origin',(0.,0.,0.));
#9107=CARTESIAN_POINT('',(-1.75,-0.85,-2.14313189850787E-16));
#9108=CARTESIAN_POINT('Origin',(0.,-0.85,0.));
#9109=CARTESIAN_POINT('',(-1.75,0.,-2.14313189850787E-16));
#9110=CARTESIAN_POINT('Origin',(1.,-0.85,0.));
#9111=CARTESIAN_POINT('',(-1.,-0.85,-1.22464679914735E-16));
#9112=CARTESIAN_POINT('Origin',(0.,-0.85,0.));
#9113=CARTESIAN_POINT('Origin',(0.,0.7,0.));
#9114=CARTESIAN_POINT('',(-1.,0.7,-1.22464679914735E-16));
#10773=UNCERTAINTY_MEASURE_WITH_UNIT(LENGTH_MEASURE(0.001),#10822,
'DISTANCE_ACCURACY_VALUE',
'Maximum model space distance between geometric entities at asserted c
onnectivities');
#10791=UNCERTAINTY_MEASURE_WITH_UNIT(LENGTH_MEASURE(0.001),#10822,
'DISTANCE_ACCURACY_VALUE',
'Maximum model space distance between geometric entities at asserted c
onnectivities');
#10803=(
GEOMETRIC_REPRESENTATION_CONTEXT(3)
GLOBAL_UNCERTAINTY_ASSIGNED_CONTEXT((#10773))
GLOBAL_UNIT_ASSIGNED_CONTEXT((#10822,#10824,#10825))
REPRESENTATION_CONTEXT('','3D')
);
#10821=(
GEOMETRIC_REPRESENTATION_CONTEXT(3)
GLOBAL_UNCERTAINTY_ASSIGNED_CONTEXT((#10791))
GLOBAL_UNIT_ASSIGNED_CONTEXT((#10822,#10824,#10825))
REPRESENTATION_CONTEXT('','3D')
);
#10822=(
LENGTH_UNIT()
NAMED_UNIT(*)
SI_UNIT(.CENTI.,.METRE.)
);
#10824=(
NAMED_UNIT(*)
PLANE_ANGLE_UNIT()
SI_UNIT($,.RADIAN.)
);
#10825=(
NAMED_UNIT(*)
SI_UNIT($,.STERADIAN.)
SOLID_ANGLE_UNIT()
);
#10837=SHAPE_DEFINITION_REPRESENTATION(#10866,#10935);
#10866=PRODUCT_DEFINITION_SHAPE('',$,#10965);
#10935=SHAPE_REPRESENTATION('',(#5990),#10803);
#10953=PRODUCT_DEFINITION_CONTEXT('part definition',#11042,'design');
#10965=PRODUCT_DEFINITION('Insert bearing','Insert bearing',#10994,#10953);
#10994=PRODUCT_DEFINITION_FORMATION('',$,#11055);
#11042=APPLICATION_CONTEXT(
'Core Data for Automotive Mechanical Design Process');
#11043=PRODUCT_CONTEXT('part definition',#11042,'mechanical');
#11055=PRODUCT('Insert bearing','Insert bearing','Insert bearing',(#11043));
#11129=COLOUR_RGB('Grey',0.48,0.52,0.57);
#11130=FILL_AREA_STYLE_COLOUR('',#11129);
#11131=FILL_AREA_STYLE('',(#11130));
#11132=SURFACE_STYLE_FILL_AREA(#11131);
#11133=SURFACE_SIDE_STYLE('',(#11132));
#11134=SURFACE_STYLE_USAGE(.BOTH.,#11133);
#11135=PRESENTATION_STYLE_ASSIGNMENT((#11134));
ENDSEC;
END-ISO-10303-21;
